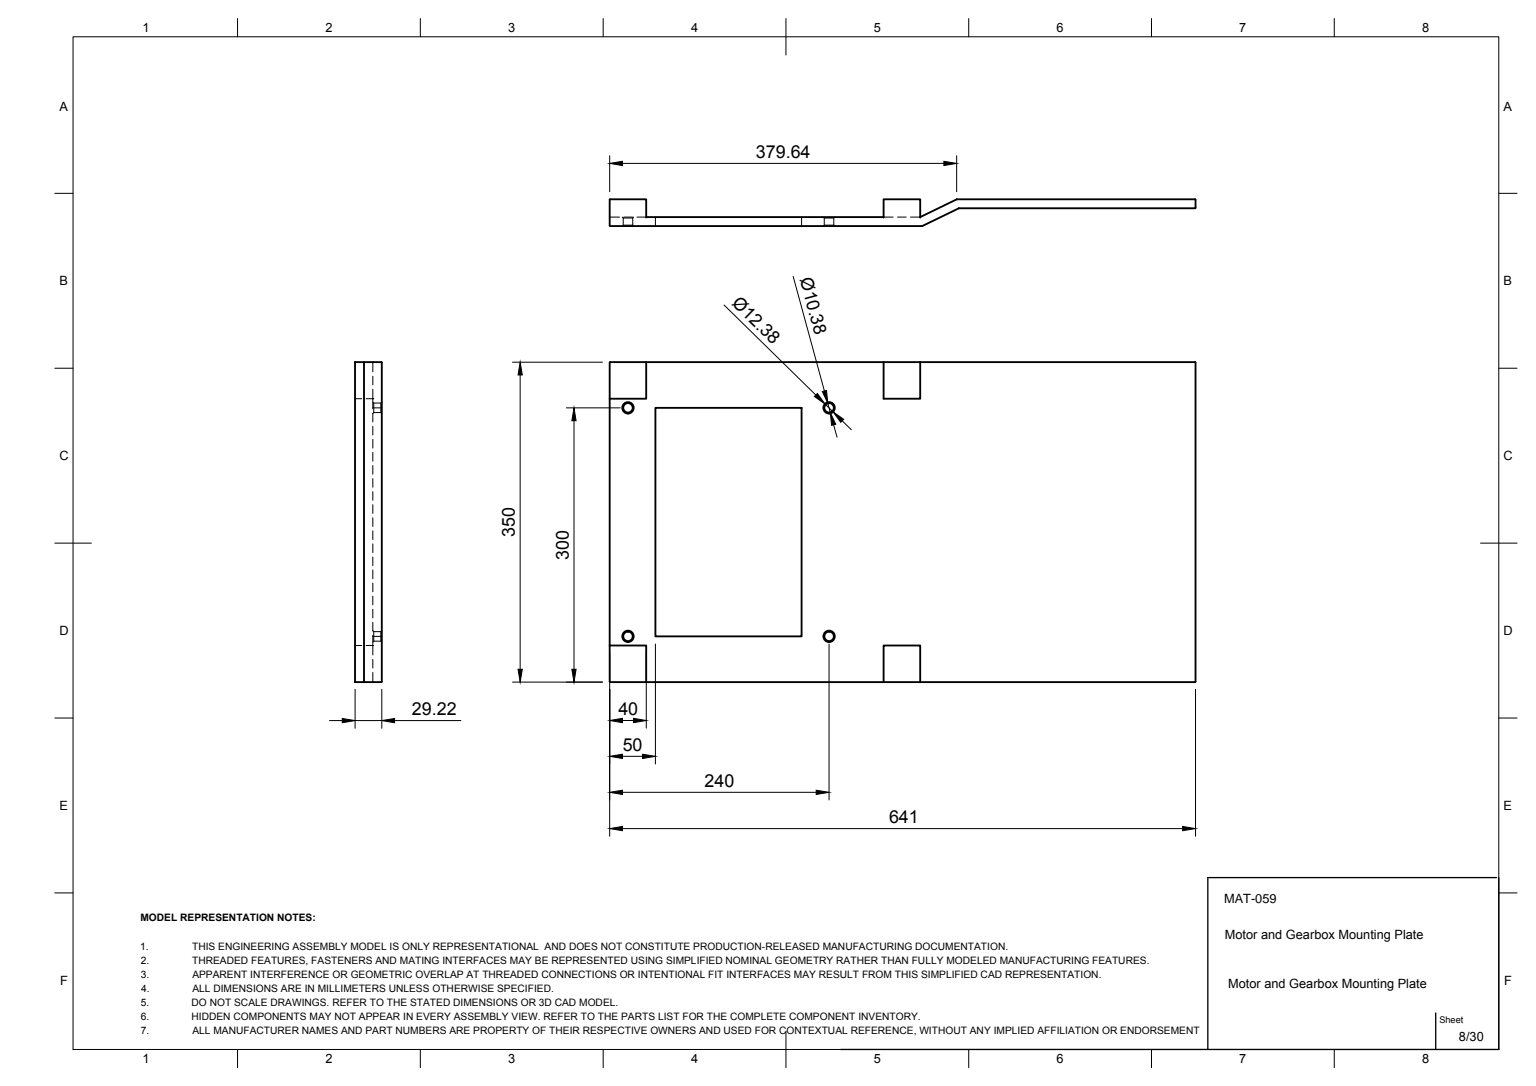
ISO-10303-21;
HEADER;
/* Generated by software containing ST-Developer
 * from STEP Tools, Inc. (www.steptools.com) 
 */

FILE_DESCRIPTION(
/* description */ ('', 'CAx-IF Rec.Pracs.---Representation and Presentation of Product Manufa
cturing Information (PMI)---4.0---2014-10-13'),
/* implementation_level */ '2;1');

FILE_NAME(
/* name */ 'Motor and Gearbox Mounting Plate.step',
/* time_stamp */ '2026-10-28T23:00:48+01:00',
/* author */ (''),
/* organization */ (''),
/* preprocessor_version */ 'ST-DEVELOPER v20.2',
/* originating_system */ 'Autodesk Translation Framework v15.17.0.0',
/* authorisation */ '');

FILE_SCHEMA (('AP242_MANAGED_MODEL_BASED_3D_ENGINEERING_MIM_LF { 1 0 10303 442 2 1 4 }'));
ENDSEC;

DATA;
#10=MECHANICAL_DESIGN_GEOMETRIC_PRESENTATION_REPRESENTATION('',(#970),#61811);
#390=ELLIPSE('',#35059,1.14442790218193,0.499999999899238);
#391=ELLIPSE('',#35060,1.14442790225741,0.499999999917943);
#392=ELLIPSE('',#35063,0.555857993550966,0.5);
#393=ELLIPSE('',#35139,0.555857993550966,0.5);
#474=B_SPLINE_SURFACE_WITH_KNOTS('',3,3,((#53444,#53445,#53446,#53447),
(#53448,#53449,#53450,#53451),(#53452,#53453,#53454,#53455),(#53456,#53457,
#53458,#53459)),.UNSPECIFIED.,.F.,.F.,.F.,(4,4),(4,4),(0.513291621409645,
1.),(-0.0253523930614869,0.),.UNSPECIFIED.);
#475=B_SPLINE_SURFACE_WITH_KNOTS('',3,3,((#53472,#53473,#53474,#53475),
(#53476,#53477,#53478,#53479),(#53480,#53481,#53482,#53483),(#53484,#53485,
#53486,#53487)),.UNSPECIFIED.,.F.,.F.,.F.,(4,4),(4,4),(0.513291621409645,
1.),(0.,0.0253730124676109),.UNSPECIFIED.);
#583=CONICAL_SURFACE('',#35152,5.68799999999971,0.785398163207466);
#584=CONICAL_SURFACE('',#35157,5.68799999999971,0.785398163337269);
#585=CONICAL_SURFACE('',#35162,5.68799999999971,0.785398163337269);
#586=CONICAL_SURFACE('',#35167,5.68799999999971,0.785398163207466);
#587=CONICAL_SURFACE('',#35172,5.688,0.785398163397448);
#588=CONICAL_SURFACE('',#35173,5.688,0.785398163397442);
#589=CONICAL_SURFACE('',#35174,5.688,0.785398163397442);
#590=CONICAL_SURFACE('',#35175,5.688,0.785398163397448);
#733=SPHERICAL_SURFACE('',#35068,0.499999999999998);
#734=SPHERICAL_SURFACE('',#35072,0.499999999999972);
#735=SPHERICAL_SURFACE('',#35076,0.499999999999972);
#736=SPHERICAL_SURFACE('',#35080,0.499999999999972);
#737=SPHERICAL_SURFACE('',#35084,0.499999999999998);
#738=SPHERICAL_SURFACE('',#35088,0.499999999999972);
#739=SPHERICAL_SURFACE('',#35101,0.5);
#740=SPHERICAL_SURFACE('',#35105,0.5);
#741=SPHERICAL_SURFACE('',#35112,0.499999999999998);
#742=SPHERICAL_SURFACE('',#35118,0.499999999999972);
#817=B_SPLINE_CURVE_WITH_KNOTS('',3,(#53461,#53462,#53463,#53464,#53465,
#53466,#53467,#53468,#53469,#53470),.UNSPECIFIED.,.F.,.F.,(4,2,2,2,4),(0.,
0.0127647979976817,0.0210777909778716,0.0238357493132096,0.025921076707915),
 .UNSPECIFIED.);
#818=B_SPLINE_CURVE_WITH_KNOTS('',3,(#53489,#53490,#53491,#53492,#53493,
#53494,#53495,#53496,#53497,#53498),.UNSPECIFIED.,.F.,.F.,(4,2,2,2,4),(0.,
0.00150625431059664,0.00349900031797075,0.00979302012528766,0.0186876936860384),
 .UNSPECIFIED.);
#896=TOROIDAL_SURFACE('',#35092,1.00000000000001,0.5);
#897=TOROIDAL_SURFACE('',#35097,1.,0.499999999999994);
#920=SHAPE_REPRESENTATION_RELATIONSHIP('SRR','None',#61978,#945);
#945=ADVANCED_BREP_SHAPE_REPRESENTATION('',(#1009),#61791);
#970=STYLED_ITEM('',(#62142),#1009);
#1009=MANIFOLD_SOLID_BREP('Body1',#33800);
#1163=CYLINDRICAL_SURFACE('',#35041,0.5);
#1164=CYLINDRICAL_SURFACE('',#35049,0.5);
#1165=CYLINDRICAL_SURFACE('',#35054,0.5);
#1166=CYLINDRICAL_SURFACE('',#35065,0.5);
#1167=CYLINDRICAL_SURFACE('',#35109,0.5);
#1168=CYLINDRICAL_SURFACE('',#35110,0.5);
#1169=CYLINDRICAL_SURFACE('',#35116,0.5);
#1170=CYLINDRICAL_SURFACE('',#35117,0.5);
#1171=CYLINDRICAL_SURFACE('',#35122,0.5);
#1172=CYLINDRICAL_SURFACE('',#35124,0.5);
#1173=CYLINDRICAL_SURFACE('',#35125,0.5);
#1174=CYLINDRICAL_SURFACE('',#35126,0.5);
#1175=CYLINDRICAL_SURFACE('',#35127,0.5);
#1176=CYLINDRICAL_SURFACE('',#35128,0.5);
#1177=CYLINDRICAL_SURFACE('',#35129,0.5);
#1178=CYLINDRICAL_SURFACE('',#35130,0.5);
#1179=CYLINDRICAL_SURFACE('',#35131,0.5);
#1180=CYLINDRICAL_SURFACE('',#35132,0.5);
#1181=CYLINDRICAL_SURFACE('',#35133,0.5);
#1182=CYLINDRICAL_SURFACE('',#35134,0.5);
#1183=CYLINDRICAL_SURFACE('',#35135,0.5);
#1184=CYLINDRICAL_SURFACE('',#35136,0.5);
#1185=CYLINDRICAL_SURFACE('',#35137,0.5);
#1186=CYLINDRICAL_SURFACE('',#35138,0.5);
#1187=CYLINDRICAL_SURFACE('',#35154,5.188);
#1188=CYLINDRICAL_SURFACE('',#35159,5.188);
#1189=CYLINDRICAL_SURFACE('',#35164,5.188);
#1190=CYLINDRICAL_SURFACE('',#35169,5.188);
#1968=FACE_BOUND('',#6698,.T.);
#1969=FACE_BOUND('',#6699,.T.);
#1970=FACE_BOUND('',#6700,.T.);
#1971=FACE_BOUND('',#6701,.T.);
#1972=FACE_BOUND('',#6702,.T.);
#1973=FACE_BOUND('',#6748,.T.);
#1974=FACE_BOUND('',#6749,.T.);
#1975=FACE_BOUND('',#6750,.T.);
#1976=FACE_BOUND('',#6751,.T.);
#1977=FACE_BOUND('',#6752,.T.);
#2674=CIRCLE('',#35042,0.5);
#2675=CIRCLE('',#35043,0.5);
#2676=CIRCLE('',#35045,6.188);
#2677=CIRCLE('',#35046,6.188);
#2678=CIRCLE('',#35047,6.188);
#2679=CIRCLE('',#35048,6.188);
#2680=CIRCLE('',#35050,0.5);
#2681=CIRCLE('',#35051,0.5);
#2682=CIRCLE('',#35053,1.00000000000015);
#2683=CIRCLE('',#35055,0.5);
#2684=CIRCLE('',#35056,0.5);
#2685=CIRCLE('',#35057,0.500000000000003);
#2686=CIRCLE('',#35058,0.499999999999992);
#2687=CIRCLE('',#35066,0.5);
#2688=CIRCLE('',#35067,0.5);
#2689=CIRCLE('',#35069,0.5);
#2690=CIRCLE('',#35070,0.499999999999998);
#2691=CIRCLE('',#35071,0.499999999999992);
#2692=CIRCLE('',#35073,0.499999999999998);
#2693=CIRCLE('',#35074,0.499999999999972);
#2694=CIRCLE('',#35075,0.499999999999996);
#2695=CIRCLE('',#35077,0.5);
#2696=CIRCLE('',#35078,0.499999999999972);
#2697=CIRCLE('',#35079,0.499999999999998);
#2698=CIRCLE('',#35081,0.499999999999972);
#2699=CIRCLE('',#35082,0.499999999999972);
#2700=CIRCLE('',#35083,0.499999999999998);
#2701=CIRCLE('',#35085,0.5);
#2702=CIRCLE('',#35086,0.499999999999998);
#2703=CIRCLE('',#35087,0.500000000000114);
#2704=CIRCLE('',#35089,0.499999999999998);
#2705=CIRCLE('',#35090,0.499999999999972);
#2706=CIRCLE('',#35091,0.499999999999972);
#2707=CIRCLE('',#35093,1.00000000000013);
#2708=CIRCLE('',#35094,0.500000000000006);
#2709=CIRCLE('',#35095,0.499999999999998);
#2710=CIRCLE('',#35096,0.5);
#2711=CIRCLE('',#35098,0.49999999999999);
#2712=CIRCLE('',#35099,0.499999999999972);
#2713=CIRCLE('',#35100,0.499999999999994);
#2714=CIRCLE('',#35102,0.5);
#2715=CIRCLE('',#35103,0.5);
#2716=CIRCLE('',#35104,0.500000000000002);
#2717=CIRCLE('',#35106,0.499999999999998);
#2718=CIRCLE('',#35107,0.5);
#2719=CIRCLE('',#35108,0.500000000000007);
#2720=CIRCLE('',#35111,0.5);
#2721=CIRCLE('',#35113,0.499999999999972);
#2722=CIRCLE('',#35114,0.499999999999998);
#2723=CIRCLE('',#35115,0.499999999999998);
#2724=CIRCLE('',#35119,0.500000000000007);
#2725=CIRCLE('',#35120,0.499999999999972);
#2726=CIRCLE('',#35121,0.500000000000003);
#2727=CIRCLE('',#35123,0.5);
#2728=CIRCLE('',#35144,6.18799999999941);
#2729=CIRCLE('',#35145,6.18799999999941);
#2730=CIRCLE('',#35146,6.18799999999941);
#2731=CIRCLE('',#35147,6.18799999999941);
#2732=CIRCLE('',#35153,5.188);
#2733=CIRCLE('',#35155,5.188);
#2734=CIRCLE('',#35156,5.188);
#2735=CIRCLE('',#35158,5.188);
#2736=CIRCLE('',#35160,5.188);
#2737=CIRCLE('',#35161,5.188);
#2738=CIRCLE('',#35163,5.188);
#2739=CIRCLE('',#35165,5.188);
#2740=CIRCLE('',#35166,5.188);
#2741=CIRCLE('',#35168,5.188);
#2742=CIRCLE('',#35170,5.188);
#2743=CIRCLE('',#35171,5.188);
#4728=FACE_OUTER_BOUND('',#6696,.T.);
#4729=FACE_OUTER_BOUND('',#6697,.T.);
#4730=FACE_OUTER_BOUND('',#6703,.T.);
#4731=FACE_OUTER_BOUND('',#6704,.T.);
#4732=FACE_OUTER_BOUND('',#6705,.T.);
#4733=FACE_OUTER_BOUND('',#6706,.T.);
#4734=FACE_OUTER_BOUND('',#6707,.T.);
#4735=FACE_OUTER_BOUND('',#6708,.T.);
#4736=FACE_OUTER_BOUND('',#6709,.T.);
#4737=FACE_OUTER_BOUND('',#6710,.T.);
#4738=FACE_OUTER_BOUND('',#6711,.T.);
#4739=FACE_OUTER_BOUND('',#6712,.T.);
#4740=FACE_OUTER_BOUND('',#6713,.T.);
#4741=FACE_OUTER_BOUND('',#6714,.T.);
#4742=FACE_OUTER_BOUND('',#6715,.T.);
#4743=FACE_OUTER_BOUND('',#6716,.T.);
#4744=FACE_OUTER_BOUND('',#6717,.T.);
#4745=FACE_OUTER_BOUND('',#6718,.T.);
#4746=FACE_OUTER_BOUND('',#6719,.T.);
#4747=FACE_OUTER_BOUND('',#6720,.T.);
#4748=FACE_OUTER_BOUND('',#6721,.T.);
#4749=FACE_OUTER_BOUND('',#6722,.T.);
#4750=FACE_OUTER_BOUND('',#6723,.T.);
#4751=FACE_OUTER_BOUND('',#6724,.T.);
#4752=FACE_OUTER_BOUND('',#6725,.T.);
#4753=FACE_OUTER_BOUND('',#6726,.T.);
#4754=FACE_OUTER_BOUND('',#6727,.T.);
#4755=FACE_OUTER_BOUND('',#6728,.T.);
#4756=FACE_OUTER_BOUND('',#6729,.T.);
#4757=FACE_OUTER_BOUND('',#6730,.T.);
#4758=FACE_OUTER_BOUND('',#6731,.T.);
#4759=FACE_OUTER_BOUND('',#6732,.T.);
#4760=FACE_OUTER_BOUND('',#6733,.T.);
#4761=FACE_OUTER_BOUND('',#6734,.T.);
#4762=FACE_OUTER_BOUND('',#6735,.T.);
#4763=FACE_OUTER_BOUND('',#6736,.T.);
#4764=FACE_OUTER_BOUND('',#6737,.T.);
#4765=FACE_OUTER_BOUND('',#6738,.T.);
#4766=FACE_OUTER_BOUND('',#6739,.T.);
#4767=FACE_OUTER_BOUND('',#6740,.T.);
#4768=FACE_OUTER_BOUND('',#6741,.T.);
#4769=FACE_OUTER_BOUND('',#6742,.T.);
#4770=FACE_OUTER_BOUND('',#6743,.T.);
#4771=FACE_OUTER_BOUND('',#6744,.T.);
#4772=FACE_OUTER_BOUND('',#6745,.T.);
#4773=FACE_OUTER_BOUND('',#6746,.T.);
#4774=FACE_OUTER_BOUND('',#6747,.T.);
#4775=FACE_OUTER_BOUND('',#6753,.T.);
#4776=FACE_OUTER_BOUND('',#6754,.T.);
#4777=FACE_OUTER_BOUND('',#6755,.T.);
#4778=FACE_OUTER_BOUND('',#6756,.T.);
#4779=FACE_OUTER_BOUND('',#6757,.T.);
#4780=FACE_OUTER_BOUND('',#6758,.T.);
#4781=FACE_OUTER_BOUND('',#6759,.T.);
#4782=FACE_OUTER_BOUND('',#6760,.T.);
#4783=FACE_OUTER_BOUND('',#6761,.T.);
#4784=FACE_OUTER_BOUND('',#6762,.T.);
#4785=FACE_OUTER_BOUND('',#6763,.T.);
#4786=FACE_OUTER_BOUND('',#6764,.T.);
#4787=FACE_OUTER_BOUND('',#6765,.T.);
#4788=FACE_OUTER_BOUND('',#6766,.T.);
#4789=FACE_OUTER_BOUND('',#6767,.T.);
#4790=FACE_OUTER_BOUND('',#6768,.T.);
#4791=FACE_OUTER_BOUND('',#6769,.T.);
#4792=FACE_OUTER_BOUND('',#6770,.T.);
#4793=FACE_OUTER_BOUND('',#6771,.T.);
#4794=FACE_OUTER_BOUND('',#6772,.T.);
#4795=FACE_OUTER_BOUND('',#6773,.T.);
#4796=FACE_OUTER_BOUND('',#6774,.T.);
#4797=FACE_OUTER_BOUND('',#6775,.T.);
#4798=FACE_OUTER_BOUND('',#6776,.T.);
#4799=FACE_OUTER_BOUND('',#6777,.T.);
#4800=FACE_OUTER_BOUND('',#6778,.T.);
#4801=FACE_OUTER_BOUND('',#6779,.T.);
#4802=FACE_OUTER_BOUND('',#6780,.T.);
#4803=FACE_OUTER_BOUND('',#6781,.T.);
#4804=FACE_OUTER_BOUND('',#6782,.T.);
#4805=FACE_OUTER_BOUND('',#6783,.T.);
#6696=EDGE_LOOP('',(#23838,#23839,#23840,#23841));
#6697=EDGE_LOOP('',(#23842,#23843,#23844,#23845,#23846,#23847,#23848,#23849,
#23850,#23851,#23852,#23853));
#6698=EDGE_LOOP('',(#23854));
#6699=EDGE_LOOP('',(#23855));
#6700=EDGE_LOOP('',(#23856,#23857,#23858,#23859));
#6701=EDGE_LOOP('',(#23860));
#6702=EDGE_LOOP('',(#23861));
#6703=EDGE_LOOP('',(#23862,#23863,#23864,#23865));
#6704=EDGE_LOOP('',(#23866,#23867,#23868,#23869,#23870,#23871,#23872,#23873,
#23874,#23875,#23876,#23877,#23878,#23879));
#6705=EDGE_LOOP('',(#23880,#23881,#23882,#23883,#23884,#23885));
#6706=EDGE_LOOP('',(#23886,#23887,#23888));
#6707=EDGE_LOOP('',(#23889,#23890,#23891));
#6708=EDGE_LOOP('',(#23892,#23893,#23894,#23895,#23896));
#6709=EDGE_LOOP('',(#23897,#23898,#23899,#23900,#23901,#23902));
#6710=EDGE_LOOP('',(#23903,#23904,#23905,#23906,#23907,#23908,#23909,#23910));
#6711=EDGE_LOOP('',(#23911,#23912,#23913,#23914));
#6712=EDGE_LOOP('',(#23915,#23916,#23917));
#6713=EDGE_LOOP('',(#23918,#23919,#23920));
#6714=EDGE_LOOP('',(#23921,#23922,#23923));
#6715=EDGE_LOOP('',(#23924,#23925,#23926));
#6716=EDGE_LOOP('',(#23927,#23928,#23929));
#6717=EDGE_LOOP('',(#23930,#23931,#23932));
#6718=EDGE_LOOP('',(#23933,#23934,#23935,#23936));
#6719=EDGE_LOOP('',(#23937,#23938,#23939,#23940));
#6720=EDGE_LOOP('',(#23941,#23942,#23943));
#6721=EDGE_LOOP('',(#23944,#23945,#23946));
#6722=EDGE_LOOP('',(#23947,#23948,#23949,#23950));
#6723=EDGE_LOOP('',(#23951,#23952,#23953,#23954));
#6724=EDGE_LOOP('',(#23955,#23956,#23957));
#6725=EDGE_LOOP('',(#23958,#23959,#23960,#23961));
#6726=EDGE_LOOP('',(#23962,#23963,#23964,#23965));
#6727=EDGE_LOOP('',(#23966,#23967,#23968));
#6728=EDGE_LOOP('',(#23969,#23970,#23971,#23972));
#6729=EDGE_LOOP('',(#23973,#23974,#23975,#23976));
#6730=EDGE_LOOP('',(#23977,#23978,#23979,#23980));
#6731=EDGE_LOOP('',(#23981,#23982,#23983,#23984));
#6732=EDGE_LOOP('',(#23985,#23986,#23987,#23988));
#6733=EDGE_LOOP('',(#23989,#23990,#23991,#23992));
#6734=EDGE_LOOP('',(#23993,#23994,#23995,#23996));
#6735=EDGE_LOOP('',(#23997,#23998,#23999,#24000));
#6736=EDGE_LOOP('',(#24001,#24002,#24003,#24004));
#6737=EDGE_LOOP('',(#24005,#24006,#24007,#24008));
#6738=EDGE_LOOP('',(#24009,#24010,#24011,#24012));
#6739=EDGE_LOOP('',(#24013,#24014,#24015,#24016));
#6740=EDGE_LOOP('',(#24017,#24018,#24019,#24020));
#6741=EDGE_LOOP('',(#24021,#24022,#24023,#24024));
#6742=EDGE_LOOP('',(#24025,#24026,#24027,#24028));
#6743=EDGE_LOOP('',(#24029,#24030,#24031,#24032));
#6744=EDGE_LOOP('',(#24033,#24034,#24035,#24036,#24037,#24038,#24039,#24040));
#6745=EDGE_LOOP('',(#24041,#24042,#24043,#24044,#24045));
#6746=EDGE_LOOP('',(#24046,#24047,#24048,#24049,#24050,#24051,#24052,#24053,
#24054,#24055,#24056,#24057,#24058,#24059));
#6747=EDGE_LOOP('',(#24060,#24061,#24062,#24063));
#6748=EDGE_LOOP('',(#24064));
#6749=EDGE_LOOP('',(#24065));
#6750=EDGE_LOOP('',(#24066,#24067,#24068,#24069));
#6751=EDGE_LOOP('',(#24070));
#6752=EDGE_LOOP('',(#24071));
#6753=EDGE_LOOP('',(#24072,#24073,#24074,#24075));
#6754=EDGE_LOOP('',(#24076,#24077,#24078,#24079));
#6755=EDGE_LOOP('',(#24080,#24081,#24082,#24083));
#6756=EDGE_LOOP('',(#24084,#24085,#24086,#24087));
#6757=EDGE_LOOP('',(#24088,#24089,#24090,#24091));
#6758=EDGE_LOOP('',(#24092,#24093,#24094,#24095,#24096));
#6759=EDGE_LOOP('',(#24097,#24098,#24099,#24100));
#6760=EDGE_LOOP('',(#24101,#24102,#24103,#24104,#24105));
#6761=EDGE_LOOP('',(#24106,#24107,#24108,#24109));
#6762=EDGE_LOOP('',(#24110,#24111,#24112,#24113,#24114));
#6763=EDGE_LOOP('',(#24115,#24116,#24117,#24118));
#6764=EDGE_LOOP('',(#24119,#24120,#24121,#24122,#24123));
#6765=EDGE_LOOP('',(#24124,#24125,#24126,#24127,#24128));
#6766=EDGE_LOOP('',(#24129,#24130,#24131,#24132,#24133));
#6767=EDGE_LOOP('',(#24134,#24135,#24136,#24137,#24138));
#6768=EDGE_LOOP('',(#24139,#24140,#24141,#24142,#24143));
#6769=EDGE_LOOP('',(#24144,#24145,#24146,#24147,#24148));
#6770=EDGE_LOOP('',(#24149,#24150,#24151,#24152,#24153));
#6771=EDGE_LOOP('',(#24154,#24155,#24156,#24157));
#6772=EDGE_LOOP('',(#24158,#24159,#24160,#24161,#24162));
#6773=EDGE_LOOP('',(#24163,#24164,#24165,#24166,#24167,#24168));
#6774=EDGE_LOOP('',(#24169,#24170,#24171,#24172,#24173));
#6775=EDGE_LOOP('',(#24174,#24175,#24176,#24177,#24178));
#6776=EDGE_LOOP('',(#24179,#24180,#24181,#24182,#24183));
#6777=EDGE_LOOP('',(#24184,#24185,#24186,#24187,#24188));
#6778=EDGE_LOOP('',(#24189,#24190,#24191,#24192));
#6779=EDGE_LOOP('',(#24193,#24194,#24195,#24196,#24197));
#6780=EDGE_LOOP('',(#24198,#24199,#24200,#24201));
#6781=EDGE_LOOP('',(#24202,#24203,#24204,#24205));
#6782=EDGE_LOOP('',(#24206,#24207,#24208,#24209));
#6783=EDGE_LOOP('',(#24210,#24211,#24212,#24213));
#8989=LINE('',#53360,#11536);
#8990=LINE('',#53363,#11537);
#8991=LINE('',#53366,#11538);
#8992=LINE('',#53368,#11539);
#8993=LINE('',#53370,#11540);
#8994=LINE('',#53372,#11541);
#8995=LINE('',#53374,#11542);
#8996=LINE('',#53376,#11543);
#8997=LINE('',#53378,#11544);
#8998=LINE('',#53380,#11545);
#8999=LINE('',#53382,#11546);
#9000=LINE('',#53384,#11547);
#9001=LINE('',#53385,#11548);
#9002=LINE('',#53392,#11549);
#9003=LINE('',#53394,#11550);
#9004=LINE('',#53396,#11551);
#9005=LINE('',#53397,#11552);
#9006=LINE('',#53406,#11553);
#9007=LINE('',#53410,#11554);
#9008=LINE('',#53412,#11555);
#9009=LINE('',#53414,#11556);
#9010=LINE('',#53416,#11557);
#9011=LINE('',#53418,#11558);
#9012=LINE('',#53420,#11559);
#9013=LINE('',#53422,#11560);
#9014=LINE('',#53424,#11561);
#9015=LINE('',#53428,#11562);
#9016=LINE('',#53430,#11563);
#9017=LINE('',#53432,#11564);
#9018=LINE('',#53433,#11565);
#9019=LINE('',#53442,#11566);
#9020=LINE('',#53502,#11567);
#9021=LINE('',#53504,#11568);
#9022=LINE('',#53505,#11569);
#9023=LINE('',#53508,#11570);
#9024=LINE('',#53510,#11571);
#9025=LINE('',#53513,#11572);
#9026=LINE('',#53515,#11573);
#9027=LINE('',#53517,#11574);
#9028=LINE('',#53518,#11575);
#9029=LINE('',#53524,#11576);
#9030=LINE('',#53592,#11577);
#9031=LINE('',#53593,#11578);
#9032=LINE('',#53598,#11579);
#9033=LINE('',#53599,#11580);
#9034=LINE('',#53607,#11581);
#9035=LINE('',#53609,#11582);
#9036=LINE('',#53610,#11583);
#9037=LINE('',#53620,#11584);
#9038=LINE('',#53622,#11585);
#9039=LINE('',#53624,#11586);
#9040=LINE('',#53625,#11587);
#9041=LINE('',#53627,#11588);
#9042=LINE('',#53628,#11589);
#9043=LINE('',#53630,#11590);
#9044=LINE('',#53632,#11591);
#9045=LINE('',#53633,#11592);
#9046=LINE('',#53635,#11593);
#9047=LINE('',#53636,#11594);
#9048=LINE('',#53638,#11595);
#9049=LINE('',#53640,#11596);
#9050=LINE('',#53641,#11597);
#9051=LINE('',#53643,#11598);
#9052=LINE('',#53644,#11599);
#9053=LINE('',#53646,#11600);
#9054=LINE('',#53648,#11601);
#9055=LINE('',#53649,#11602);
#9056=LINE('',#53651,#11603);
#9057=LINE('',#53652,#11604);
#9058=LINE('',#53655,#11605);
#9059=LINE('',#53659,#11606);
#9060=LINE('',#53662,#11607);
#9061=LINE('',#53663,#11608);
#9062=LINE('',#53665,#11609);
#9063=LINE('',#53666,#11610);
#9064=LINE('',#53669,#11611);
#9065=LINE('',#53671,#11612);
#9066=LINE('',#53672,#11613);
#9067=LINE('',#53674,#11614);
#9068=LINE('',#53676,#11615);
#9069=LINE('',#53678,#11616);
#9070=LINE('',#53679,#11617);
#9071=LINE('',#53687,#11618);
#9072=LINE('',#53689,#11619);
#9073=LINE('',#53691,#11620);
#9074=LINE('',#53692,#11621);
#9075=LINE('',#53704,#11622);
#9076=LINE('',#53707,#11623);
#9077=LINE('',#53714,#11624);
#9078=LINE('',#53717,#11625);
#9079=LINE('',#53724,#11626);
#9080=LINE('',#53727,#11627);
#9081=LINE('',#53734,#11628);
#9082=LINE('',#53737,#11629);
#9083=LINE('',#53742,#11630);
#9084=LINE('',#53744,#11631);
#9085=LINE('',#53746,#11632);
#9086=LINE('',#53748,#11633);
#9087=LINE('',#53750,#11634);
#9088=LINE('',#53754,#11635);
#9089=LINE('',#53756,#11636);
#9090=LINE('',#53757,#11637);
#9091=LINE('',#53759,#11638);
#9092=LINE('',#53761,#11639);
#9093=LINE('',#53765,#11640);
#9094=LINE('',#53766,#11641);
#9095=LINE('',#53768,#11642);
#9096=LINE('',#53771,#11643);
#9097=LINE('',#53774,#11644);
#9098=LINE('',#53775,#11645);
#9099=LINE('',#53777,#11646);
#9100=LINE('',#53779,#11647);
#11536=VECTOR('',#40671,10.);
#11537=VECTOR('',#40674,10.);
#11538=VECTOR('',#40677,10.);
#11539=VECTOR('',#40678,10.);
#11540=VECTOR('',#40679,10.);
#11541=VECTOR('',#40680,10.);
#11542=VECTOR('',#40681,10.);
#11543=VECTOR('',#40682,10.);
#11544=VECTOR('',#40683,10.);
#11545=VECTOR('',#40684,10.);
#11546=VECTOR('',#40685,10.);
#11547=VECTOR('',#40686,10.);
#11548=VECTOR('',#40687,10.);
#11549=VECTOR('',#40692,10.);
#11550=VECTOR('',#40693,10.);
#11551=VECTOR('',#40694,10.);
#11552=VECTOR('',#40695,10.);
#11553=VECTOR('',#40704,10.);
#11554=VECTOR('',#40709,10.);
#11555=VECTOR('',#40710,10.);
#11556=VECTOR('',#40711,10.);
#11557=VECTOR('',#40712,10.);
#11558=VECTOR('',#40713,10.);
#11559=VECTOR('',#40714,10.);
#11560=VECTOR('',#40715,10.);
#11561=VECTOR('',#40716,10.);
#11562=VECTOR('',#40719,10.);
#11563=VECTOR('',#40720,10.);
#11564=VECTOR('',#40721,10.);
#11565=VECTOR('',#40722,10.);
#11566=VECTOR('',#40731,10.);
#11567=VECTOR('',#40740,10.);
#11568=VECTOR('',#40741,10.);
#11569=VECTOR('',#40742,10.);
#11570=VECTOR('',#40745,10.);
#11571=VECTOR('',#40748,10.);
#11572=VECTOR('',#40751,10.);
#11573=VECTOR('',#40752,10.);
#11574=VECTOR('',#40753,10.);
#11575=VECTOR('',#40754,10.);
#11576=VECTOR('',#40761,10.);
#11577=VECTOR('',#40846,10.);
#11578=VECTOR('',#40847,10.);
#11579=VECTOR('',#40852,10.);
#11580=VECTOR('',#40853,10.);
#11581=VECTOR('',#40864,10.);
#11582=VECTOR('',#40867,10.);
#11583=VECTOR('',#40868,10.);
#11584=VECTOR('',#40881,10.);
#11585=VECTOR('',#40884,10.);
#11586=VECTOR('',#40887,10.);
#11587=VECTOR('',#40888,10.);
#11588=VECTOR('',#40891,10.);
#11589=VECTOR('',#40892,10.);
#11590=VECTOR('',#40895,10.);
#11591=VECTOR('',#40898,10.);
#11592=VECTOR('',#40899,10.);
#11593=VECTOR('',#40902,10.);
#11594=VECTOR('',#40903,10.);
#11595=VECTOR('',#40906,10.);
#11596=VECTOR('',#40909,10.);
#11597=VECTOR('',#40910,10.);
#11598=VECTOR('',#40913,10.);
#11599=VECTOR('',#40914,10.);
#11600=VECTOR('',#40917,10.);
#11601=VECTOR('',#40920,10.);
#11602=VECTOR('',#40921,10.);
#11603=VECTOR('',#40924,10.);
#11604=VECTOR('',#40925,10.);
#11605=VECTOR('',#40930,10.);
#11606=VECTOR('',#40935,10.);
#11607=VECTOR('',#40938,10.);
#11608=VECTOR('',#40939,10.);
#11609=VECTOR('',#40940,10.);
#11610=VECTOR('',#40941,10.);
#11611=VECTOR('',#40944,10.);
#11612=VECTOR('',#40945,10.);
#11613=VECTOR('',#40946,10.);
#11614=VECTOR('',#40949,10.);
#11615=VECTOR('',#40950,10.);
#11616=VECTOR('',#40951,10.);
#11617=VECTOR('',#40952,10.);
#11618=VECTOR('',#40959,10.);
#11619=VECTOR('',#40960,10.);
#11620=VECTOR('',#40961,10.);
#11621=VECTOR('',#40962,10.);
#11622=VECTOR('',#40979,5.68799999999971);
#11623=VECTOR('',#40982,5.188);
#11624=VECTOR('',#40991,5.68799999999971);
#11625=VECTOR('',#40994,5.188);
#11626=VECTOR('',#41003,5.68799999999971);
#11627=VECTOR('',#41006,5.188);
#11628=VECTOR('',#41015,5.68799999999971);
#11629=VECTOR('',#41018,5.188);
#11630=VECTOR('',#41025,5.688);
#11631=VECTOR('',#41028,5.688);
#11632=VECTOR('',#41031,5.688);
#11633=VECTOR('',#41034,5.688);
#11634=VECTOR('',#41037,10.);
#11635=VECTOR('',#41042,10.);
#11636=VECTOR('',#41043,10.);
#11637=VECTOR('',#41044,10.);
#11638=VECTOR('',#41047,10.);
#11639=VECTOR('',#41050,10.);
#11640=VECTOR('',#41055,10.);
#11641=VECTOR('',#41056,10.);
#11642=VECTOR('',#41059,10.);
#11643=VECTOR('',#41064,10.);
#11644=VECTOR('',#41069,10.);
#11645=VECTOR('',#41070,10.);
#11646=VECTOR('',#41073,10.);
#11647=VECTOR('',#41076,10.);
#14210=VERTEX_POINT('',#53356);
#14211=VERTEX_POINT('',#53357);
#14212=VERTEX_POINT('',#53359);
#14213=VERTEX_POINT('',#53361);
#14214=VERTEX_POINT('',#53365);
#14215=VERTEX_POINT('',#53367);
#14216=VERTEX_POINT('',#53369);
#14217=VERTEX_POINT('',#53371);
#14218=VERTEX_POINT('',#53373);
#14219=VERTEX_POINT('',#53375);
#14220=VERTEX_POINT('',#53377);
#14221=VERTEX_POINT('',#53379);
#14222=VERTEX_POINT('',#53381);
#14223=VERTEX_POINT('',#53383);
#14224=VERTEX_POINT('',#53386);
#14225=VERTEX_POINT('',#53388);
#14226=VERTEX_POINT('',#53390);
#14227=VERTEX_POINT('',#53391);
#14228=VERTEX_POINT('',#53393);
#14229=VERTEX_POINT('',#53395);
#14230=VERTEX_POINT('',#53398);
#14231=VERTEX_POINT('',#53400);
#14232=VERTEX_POINT('',#53403);
#14233=VERTEX_POINT('',#53405);
#14234=VERTEX_POINT('',#53409);
#14235=VERTEX_POINT('',#53411);
#14236=VERTEX_POINT('',#53413);
#14237=VERTEX_POINT('',#53415);
#14238=VERTEX_POINT('',#53417);
#14239=VERTEX_POINT('',#53419);
#14240=VERTEX_POINT('',#53421);
#14241=VERTEX_POINT('',#53423);
#14242=VERTEX_POINT('',#53425);
#14243=VERTEX_POINT('',#53427);
#14244=VERTEX_POINT('',#53429);
#14245=VERTEX_POINT('',#53431);
#14246=VERTEX_POINT('',#53435);
#14247=VERTEX_POINT('',#53437);
#14248=VERTEX_POINT('',#53439);
#14249=VERTEX_POINT('',#53441);
#14250=VERTEX_POINT('',#53460);
#14251=VERTEX_POINT('',#53488);
#14252=VERTEX_POINT('',#53501);
#14253=VERTEX_POINT('',#53503);
#14254=VERTEX_POINT('',#53507);
#14255=VERTEX_POINT('',#53512);
#14256=VERTEX_POINT('',#53514);
#14257=VERTEX_POINT('',#53516);
#14258=VERTEX_POINT('',#53520);
#14259=VERTEX_POINT('',#53522);
#14260=VERTEX_POINT('',#53526);
#14261=VERTEX_POINT('',#53528);
#14262=VERTEX_POINT('',#53532);
#14263=VERTEX_POINT('',#53537);
#14264=VERTEX_POINT('',#53538);
#14265=VERTEX_POINT('',#53540);
#14266=VERTEX_POINT('',#53544);
#14267=VERTEX_POINT('',#53545);
#14268=VERTEX_POINT('',#53550);
#14269=VERTEX_POINT('',#53551);
#14270=VERTEX_POINT('',#53553);
#14271=VERTEX_POINT('',#53557);
#14272=VERTEX_POINT('',#53558);
#14273=VERTEX_POINT('',#53563);
#14274=VERTEX_POINT('',#53564);
#14275=VERTEX_POINT('',#53566);
#14276=VERTEX_POINT('',#53568);
#14277=VERTEX_POINT('',#53572);
#14278=VERTEX_POINT('',#53573);
#14279=VERTEX_POINT('',#53578);
#14280=VERTEX_POINT('',#53579);
#14281=VERTEX_POINT('',#53581);
#14282=VERTEX_POINT('',#53585);
#14283=VERTEX_POINT('',#53586);
#14284=VERTEX_POINT('',#53588);
#14285=VERTEX_POINT('',#53595);
#14286=VERTEX_POINT('',#53596);
#14287=VERTEX_POINT('',#53601);
#14288=VERTEX_POINT('',#53603);
#14289=VERTEX_POINT('',#53612);
#14290=VERTEX_POINT('',#53613);
#14291=VERTEX_POINT('',#53618);
#14292=VERTEX_POINT('',#53657);
#14293=VERTEX_POINT('',#53661);
#14294=VERTEX_POINT('',#53664);
#14295=VERTEX_POINT('',#53668);
#14296=VERTEX_POINT('',#53670);
#14297=VERTEX_POINT('',#53675);
#14298=VERTEX_POINT('',#53677);
#14299=VERTEX_POINT('',#53681);
#14300=VERTEX_POINT('',#53683);
#14301=VERTEX_POINT('',#53685);
#14302=VERTEX_POINT('',#53686);
#14303=VERTEX_POINT('',#53688);
#14304=VERTEX_POINT('',#53690);
#14305=VERTEX_POINT('',#53693);
#14306=VERTEX_POINT('',#53695);
#14307=VERTEX_POINT('',#53702);
#14308=VERTEX_POINT('',#53706);
#14309=VERTEX_POINT('',#53708);
#14310=VERTEX_POINT('',#53712);
#14311=VERTEX_POINT('',#53716);
#14312=VERTEX_POINT('',#53718);
#14313=VERTEX_POINT('',#53722);
#14314=VERTEX_POINT('',#53726);
#14315=VERTEX_POINT('',#53728);
#14316=VERTEX_POINT('',#53732);
#14317=VERTEX_POINT('',#53736);
#14318=VERTEX_POINT('',#53738);
#14319=VERTEX_POINT('',#53753);
#14320=VERTEX_POINT('',#53755);
#14321=VERTEX_POINT('',#53764);
#17821=EDGE_CURVE('',#14210,#14211,#2674,.F.);
#17822=EDGE_CURVE('',#14211,#14212,#8989,.T.);
#17823=EDGE_CURVE('',#14212,#14213,#2675,.F.);
#17824=EDGE_CURVE('',#14213,#14210,#8990,.T.);
#17825=EDGE_CURVE('',#14211,#14214,#8991,.T.);
#17826=EDGE_CURVE('',#14214,#14215,#8992,.T.);
#17827=EDGE_CURVE('',#14216,#14215,#8993,.T.);
#17828=EDGE_CURVE('',#14216,#14217,#8994,.T.);
#17829=EDGE_CURVE('',#14217,#14218,#8995,.T.);
#17830=EDGE_CURVE('',#14219,#14218,#8996,.T.);
#17831=EDGE_CURVE('',#14219,#14220,#8997,.T.);
#17832=EDGE_CURVE('',#14220,#14221,#8998,.T.);
#17833=EDGE_CURVE('',#14222,#14221,#8999,.T.);
#17834=EDGE_CURVE('',#14222,#14223,#9000,.T.);
#17835=EDGE_CURVE('',#14223,#14212,#9001,.T.);
#17836=EDGE_CURVE('',#14224,#14224,#2676,.T.);
#17837=EDGE_CURVE('',#14225,#14225,#2677,.T.);
#17838=EDGE_CURVE('',#14226,#14227,#9002,.T.);
#17839=EDGE_CURVE('',#14227,#14228,#9003,.T.);
#17840=EDGE_CURVE('',#14228,#14229,#9004,.T.);
#17841=EDGE_CURVE('',#14229,#14226,#9005,.T.);
#17842=EDGE_CURVE('',#14230,#14230,#2678,.T.);
#17843=EDGE_CURVE('',#14231,#14231,#2679,.T.);
#17844=EDGE_CURVE('',#14221,#14232,#2680,.F.);
#17845=EDGE_CURVE('',#14232,#14233,#9006,.T.);
#17846=EDGE_CURVE('',#14233,#14222,#2681,.F.);
#17847=EDGE_CURVE('',#14233,#14234,#9007,.T.);
#17848=EDGE_CURVE('',#14232,#14235,#9008,.T.);
#17849=EDGE_CURVE('',#14235,#14236,#9009,.T.);
#17850=EDGE_CURVE('',#14237,#14236,#9010,.T.);
#17851=EDGE_CURVE('',#14238,#14237,#9011,.T.);
#17852=EDGE_CURVE('',#14239,#14238,#9012,.T.);
#17853=EDGE_CURVE('',#14240,#14239,#9013,.T.);
#17854=EDGE_CURVE('',#14241,#14240,#9014,.T.);
#17855=EDGE_CURVE('',#14242,#14241,#2682,.T.);
#17856=EDGE_CURVE('',#14243,#14242,#9015,.T.);
#17857=EDGE_CURVE('',#14244,#14243,#9016,.T.);
#17858=EDGE_CURVE('',#14245,#14244,#9017,.T.);
#17859=EDGE_CURVE('',#14245,#14234,#9018,.T.);
#17860=EDGE_CURVE('',#14219,#14246,#2683,.T.);
#17861=EDGE_CURVE('',#14247,#14218,#2684,.T.);
#17862=EDGE_CURVE('',#14247,#14248,#2685,.T.);
#17863=EDGE_CURVE('',#14248,#14249,#9019,.T.);
#17864=EDGE_CURVE('',#14249,#14246,#2686,.T.);
#17865=EDGE_CURVE('',#14250,#14247,#817,.T.);
#17866=EDGE_CURVE('',#14250,#14248,#390,.T.);
#17867=EDGE_CURVE('',#14246,#14251,#818,.T.);
#17868=EDGE_CURVE('',#14249,#14251,#391,.T.);
#17869=EDGE_CURVE('',#14246,#14252,#9020,.T.);
#17870=EDGE_CURVE('',#14252,#14253,#9021,.T.);
#17871=EDGE_CURVE('',#14220,#14253,#9022,.T.);
#17872=EDGE_CURVE('',#14251,#14254,#9023,.T.);
#17873=EDGE_CURVE('',#14237,#14254,#392,.F.);
#17874=EDGE_CURVE('',#14236,#14252,#9024,.T.);
#17875=EDGE_CURVE('',#14255,#14250,#9025,.T.);
#17876=EDGE_CURVE('',#14256,#14255,#9026,.T.);
#17877=EDGE_CURVE('',#14257,#14256,#9027,.T.);
#17878=EDGE_CURVE('',#14254,#14257,#9028,.T.);
#17879=EDGE_CURVE('',#14258,#14216,#2687,.F.);
#17880=EDGE_CURVE('',#14215,#14259,#2688,.F.);
#17881=EDGE_CURVE('',#14259,#14258,#9029,.T.);
#17882=EDGE_CURVE('',#14260,#14256,#2689,.F.);
#17883=EDGE_CURVE('',#14261,#14260,#2690,.F.);
#17884=EDGE_CURVE('',#14256,#14261,#2691,.F.);
#17885=EDGE_CURVE('',#14262,#14257,#2692,.F.);
#17886=EDGE_CURVE('',#14238,#14262,#2693,.F.);
#17887=EDGE_CURVE('',#14257,#14238,#2694,.F.);
#17888=EDGE_CURVE('',#14263,#14264,#2695,.F.);
#17889=EDGE_CURVE('',#14265,#14263,#2696,.F.);
#17890=EDGE_CURVE('',#14264,#14265,#2697,.F.);
#17891=EDGE_CURVE('',#14266,#14267,#2698,.F.);
#17892=EDGE_CURVE('',#14239,#14266,#2699,.F.);
#17893=EDGE_CURVE('',#14267,#14239,#2700,.F.);
#17894=EDGE_CURVE('',#14268,#14269,#2701,.F.);
#17895=EDGE_CURVE('',#14270,#14268,#2702,.F.);
#17896=EDGE_CURVE('',#14269,#14270,#2703,.F.);
#17897=EDGE_CURVE('',#14271,#14272,#2704,.F.);
#17898=EDGE_CURVE('',#14240,#14271,#2705,.F.);
#17899=EDGE_CURVE('',#14272,#14240,#2706,.F.);
#17900=EDGE_CURVE('',#14273,#14274,#2707,.T.);
#17901=EDGE_CURVE('',#14275,#14274,#2708,.T.);
#17902=EDGE_CURVE('',#14276,#14275,#2709,.F.);
#17903=EDGE_CURVE('',#14273,#14276,#2710,.T.);
#17904=EDGE_CURVE('',#14277,#14278,#2711,.F.);
#17905=EDGE_CURVE('',#14242,#14277,#2712,.T.);
#17906=EDGE_CURVE('',#14278,#14241,#2713,.T.);
#17907=EDGE_CURVE('',#14279,#14280,#2714,.F.);
#17908=EDGE_CURVE('',#14281,#14279,#2715,.F.);
#17909=EDGE_CURVE('',#14280,#14281,#2716,.F.);
#17910=EDGE_CURVE('',#14282,#14283,#2717,.F.);
#17911=EDGE_CURVE('',#14284,#14282,#2718,.F.);
#17912=EDGE_CURVE('',#14283,#14284,#2719,.F.);
#17913=EDGE_CURVE('',#14279,#14284,#9030,.T.);
#17914=EDGE_CURVE('',#14282,#14281,#9031,.T.);
#17915=EDGE_CURVE('',#14285,#14286,#2720,.T.);
#17916=EDGE_CURVE('',#14286,#14283,#9032,.T.);
#17917=EDGE_CURVE('',#14284,#14285,#9033,.T.);
#17918=EDGE_CURVE('',#14243,#14287,#2721,.F.);
#17919=EDGE_CURVE('',#14288,#14243,#2722,.F.);
#17920=EDGE_CURVE('',#14287,#14288,#2723,.F.);
#17921=EDGE_CURVE('',#14277,#14288,#9034,.T.);
#17922=EDGE_CURVE('',#14288,#14280,#9035,.T.);
#17923=EDGE_CURVE('',#14281,#14287,#9036,.T.);
#17924=EDGE_CURVE('',#14289,#14290,#2724,.F.);
#17925=EDGE_CURVE('',#14244,#14289,#2725,.F.);
#17926=EDGE_CURVE('',#14290,#14244,#2726,.F.);
#17927=EDGE_CURVE('',#14291,#14245,#2727,.T.);
#17928=EDGE_CURVE('',#14289,#14291,#9037,.T.);
#17929=EDGE_CURVE('',#14287,#14290,#9038,.T.);
#17930=EDGE_CURVE('',#14290,#14282,#9039,.T.);
#17931=EDGE_CURVE('',#14283,#14289,#9040,.T.);
#17932=EDGE_CURVE('',#14274,#14279,#9041,.T.);
#17933=EDGE_CURVE('',#14280,#14275,#9042,.T.);
#17934=EDGE_CURVE('',#14271,#14278,#9043,.T.);
#17935=EDGE_CURVE('',#14278,#14276,#9044,.T.);
#17936=EDGE_CURVE('',#14275,#14277,#9045,.T.);
#17937=EDGE_CURVE('',#14268,#14273,#9046,.T.);
#17938=EDGE_CURVE('',#14276,#14270,#9047,.T.);
#17939=EDGE_CURVE('',#14266,#14272,#9048,.T.);
#17940=EDGE_CURVE('',#14272,#14269,#9049,.T.);
#17941=EDGE_CURVE('',#14270,#14271,#9050,.T.);
#17942=EDGE_CURVE('',#14263,#14268,#9051,.T.);
#17943=EDGE_CURVE('',#14269,#14265,#9052,.T.);
#17944=EDGE_CURVE('',#14262,#14267,#9053,.T.);
#17945=EDGE_CURVE('',#14267,#14264,#9054,.T.);
#17946=EDGE_CURVE('',#14265,#14266,#9055,.T.);
#17947=EDGE_CURVE('',#14260,#14263,#9056,.T.);
#17948=EDGE_CURVE('',#14264,#14261,#9057,.T.);
#17949=EDGE_CURVE('',#14261,#14262,#9058,.T.);
#17950=EDGE_CURVE('',#14255,#14292,#393,.F.);
#17951=EDGE_CURVE('',#14292,#14260,#9059,.T.);
#17952=EDGE_CURVE('',#14213,#14293,#9060,.T.);
#17953=EDGE_CURVE('',#14293,#14291,#9061,.T.);
#17954=EDGE_CURVE('',#14286,#14294,#9062,.T.);
#17955=EDGE_CURVE('',#14210,#14294,#9063,.T.);
#17956=EDGE_CURVE('',#14295,#14285,#9064,.T.);
#17957=EDGE_CURVE('',#14296,#14295,#9065,.T.);
#17958=EDGE_CURVE('',#14294,#14296,#9066,.T.);
#17959=EDGE_CURVE('',#14259,#14295,#9067,.T.);
#17960=EDGE_CURVE('',#14292,#14297,#9068,.T.);
#17961=EDGE_CURVE('',#14297,#14298,#9069,.T.);
#17962=EDGE_CURVE('',#14258,#14298,#9070,.T.);
#17963=EDGE_CURVE('',#14299,#14299,#2728,.T.);
#17964=EDGE_CURVE('',#14300,#14300,#2729,.T.);
#17965=EDGE_CURVE('',#14301,#14302,#9071,.T.);
#17966=EDGE_CURVE('',#14302,#14303,#9072,.T.);
#17967=EDGE_CURVE('',#14303,#14304,#9073,.T.);
#17968=EDGE_CURVE('',#14304,#14301,#9074,.T.);
#17969=EDGE_CURVE('',#14305,#14305,#2730,.T.);
#17970=EDGE_CURVE('',#14306,#14306,#2731,.T.);
#17971=EDGE_CURVE('',#14307,#14307,#2732,.T.);
#17972=EDGE_CURVE('',#14307,#14299,#9075,.T.);
#17973=EDGE_CURVE('',#14307,#14308,#9076,.T.);
#17974=EDGE_CURVE('',#14309,#14308,#2733,.T.);
#17975=EDGE_CURVE('',#14308,#14309,#2734,.T.);
#17976=EDGE_CURVE('',#14310,#14310,#2735,.T.);
#17977=EDGE_CURVE('',#14310,#14306,#9077,.T.);
#17978=EDGE_CURVE('',#14310,#14311,#9078,.T.);
#17979=EDGE_CURVE('',#14312,#14311,#2736,.T.);
#17980=EDGE_CURVE('',#14311,#14312,#2737,.T.);
#17981=EDGE_CURVE('',#14313,#14313,#2738,.T.);
#17982=EDGE_CURVE('',#14313,#14300,#9079,.T.);
#17983=EDGE_CURVE('',#14313,#14314,#9080,.T.);
#17984=EDGE_CURVE('',#14315,#14314,#2739,.T.);
#17985=EDGE_CURVE('',#14314,#14315,#2740,.T.);
#17986=EDGE_CURVE('',#14316,#14316,#2741,.T.);
#17987=EDGE_CURVE('',#14316,#14305,#9081,.T.);
#17988=EDGE_CURVE('',#14316,#14317,#9082,.T.);
#17989=EDGE_CURVE('',#14318,#14317,#2742,.T.);
#17990=EDGE_CURVE('',#14317,#14318,#2743,.T.);
#17991=EDGE_CURVE('',#14309,#14231,#9083,.T.);
#17992=EDGE_CURVE('',#14312,#14224,#9084,.T.);
#17993=EDGE_CURVE('',#14315,#14230,#9085,.T.);
#17994=EDGE_CURVE('',#14318,#14225,#9086,.T.);
#17995=EDGE_CURVE('',#14214,#14296,#9087,.T.);
#17996=EDGE_CURVE('',#14319,#14297,#9088,.T.);
#17997=EDGE_CURVE('',#14320,#14319,#9089,.T.);
#17998=EDGE_CURVE('',#14298,#14320,#9090,.T.);
#17999=EDGE_CURVE('',#14217,#14320,#9091,.T.);
#18000=EDGE_CURVE('',#14247,#14319,#9092,.T.);
#18001=EDGE_CURVE('',#14321,#14293,#9093,.T.);
#18002=EDGE_CURVE('',#14223,#14321,#9094,.T.);
#18003=EDGE_CURVE('',#14234,#14321,#9095,.T.);
#18004=EDGE_CURVE('',#14253,#14235,#9096,.T.);
#18005=EDGE_CURVE('',#14228,#14304,#9097,.T.);
#18006=EDGE_CURVE('',#14303,#14229,#9098,.T.);
#18007=EDGE_CURVE('',#14226,#14302,#9099,.T.);
#18008=EDGE_CURVE('',#14227,#14301,#9100,.T.);
#23838=ORIENTED_EDGE('',*,*,#17821,.T.);
#23839=ORIENTED_EDGE('',*,*,#17822,.T.);
#23840=ORIENTED_EDGE('',*,*,#17823,.T.);
#23841=ORIENTED_EDGE('',*,*,#17824,.T.);
#23842=ORIENTED_EDGE('',*,*,#17822,.F.);
#23843=ORIENTED_EDGE('',*,*,#17825,.T.);
#23844=ORIENTED_EDGE('',*,*,#17826,.T.);
#23845=ORIENTED_EDGE('',*,*,#17827,.F.);
#23846=ORIENTED_EDGE('',*,*,#17828,.T.);
#23847=ORIENTED_EDGE('',*,*,#17829,.T.);
#23848=ORIENTED_EDGE('',*,*,#17830,.F.);
#23849=ORIENTED_EDGE('',*,*,#17831,.T.);
#23850=ORIENTED_EDGE('',*,*,#17832,.T.);
#23851=ORIENTED_EDGE('',*,*,#17833,.F.);
#23852=ORIENTED_EDGE('',*,*,#17834,.T.);
#23853=ORIENTED_EDGE('',*,*,#17835,.T.);
#23854=ORIENTED_EDGE('',*,*,#17836,.F.);
#23855=ORIENTED_EDGE('',*,*,#17837,.F.);
#23856=ORIENTED_EDGE('',*,*,#17838,.T.);
#23857=ORIENTED_EDGE('',*,*,#17839,.T.);
#23858=ORIENTED_EDGE('',*,*,#17840,.T.);
#23859=ORIENTED_EDGE('',*,*,#17841,.T.);
#23860=ORIENTED_EDGE('',*,*,#17842,.F.);
#23861=ORIENTED_EDGE('',*,*,#17843,.F.);
#23862=ORIENTED_EDGE('',*,*,#17844,.T.);
#23863=ORIENTED_EDGE('',*,*,#17845,.T.);
#23864=ORIENTED_EDGE('',*,*,#17846,.T.);
#23865=ORIENTED_EDGE('',*,*,#17833,.T.);
#23866=ORIENTED_EDGE('',*,*,#17847,.F.);
#23867=ORIENTED_EDGE('',*,*,#17845,.F.);
#23868=ORIENTED_EDGE('',*,*,#17848,.T.);
#23869=ORIENTED_EDGE('',*,*,#17849,.T.);
#23870=ORIENTED_EDGE('',*,*,#17850,.F.);
#23871=ORIENTED_EDGE('',*,*,#17851,.F.);
#23872=ORIENTED_EDGE('',*,*,#17852,.F.);
#23873=ORIENTED_EDGE('',*,*,#17853,.F.);
#23874=ORIENTED_EDGE('',*,*,#17854,.F.);
#23875=ORIENTED_EDGE('',*,*,#17855,.F.);
#23876=ORIENTED_EDGE('',*,*,#17856,.F.);
#23877=ORIENTED_EDGE('',*,*,#17857,.F.);
#23878=ORIENTED_EDGE('',*,*,#17858,.F.);
#23879=ORIENTED_EDGE('',*,*,#17859,.T.);
#23880=ORIENTED_EDGE('',*,*,#17860,.F.);
#23881=ORIENTED_EDGE('',*,*,#17830,.T.);
#23882=ORIENTED_EDGE('',*,*,#17861,.F.);
#23883=ORIENTED_EDGE('',*,*,#17862,.T.);
#23884=ORIENTED_EDGE('',*,*,#17863,.T.);
#23885=ORIENTED_EDGE('',*,*,#17864,.T.);
#23886=ORIENTED_EDGE('',*,*,#17865,.F.);
#23887=ORIENTED_EDGE('',*,*,#17866,.T.);
#23888=ORIENTED_EDGE('',*,*,#17862,.F.);
#23889=ORIENTED_EDGE('',*,*,#17867,.F.);
#23890=ORIENTED_EDGE('',*,*,#17864,.F.);
#23891=ORIENTED_EDGE('',*,*,#17868,.T.);
#23892=ORIENTED_EDGE('',*,*,#17860,.T.);
#23893=ORIENTED_EDGE('',*,*,#17869,.T.);
#23894=ORIENTED_EDGE('',*,*,#17870,.T.);
#23895=ORIENTED_EDGE('',*,*,#17871,.F.);
#23896=ORIENTED_EDGE('',*,*,#17831,.F.);
#23897=ORIENTED_EDGE('',*,*,#17867,.T.);
#23898=ORIENTED_EDGE('',*,*,#17872,.T.);
#23899=ORIENTED_EDGE('',*,*,#17873,.F.);
#23900=ORIENTED_EDGE('',*,*,#17850,.T.);
#23901=ORIENTED_EDGE('',*,*,#17874,.T.);
#23902=ORIENTED_EDGE('',*,*,#17869,.F.);
#23903=ORIENTED_EDGE('',*,*,#17868,.F.);
#23904=ORIENTED_EDGE('',*,*,#17863,.F.);
#23905=ORIENTED_EDGE('',*,*,#17866,.F.);
#23906=ORIENTED_EDGE('',*,*,#17875,.F.);
#23907=ORIENTED_EDGE('',*,*,#17876,.F.);
#23908=ORIENTED_EDGE('',*,*,#17877,.F.);
#23909=ORIENTED_EDGE('',*,*,#17878,.F.);
#23910=ORIENTED_EDGE('',*,*,#17872,.F.);
#23911=ORIENTED_EDGE('',*,*,#17879,.T.);
#23912=ORIENTED_EDGE('',*,*,#17827,.T.);
#23913=ORIENTED_EDGE('',*,*,#17880,.T.);
#23914=ORIENTED_EDGE('',*,*,#17881,.T.);
#23915=ORIENTED_EDGE('',*,*,#17882,.F.);
#23916=ORIENTED_EDGE('',*,*,#17883,.F.);
#23917=ORIENTED_EDGE('',*,*,#17884,.F.);
#23918=ORIENTED_EDGE('',*,*,#17885,.F.);
#23919=ORIENTED_EDGE('',*,*,#17886,.F.);
#23920=ORIENTED_EDGE('',*,*,#17887,.F.);
#23921=ORIENTED_EDGE('',*,*,#17888,.F.);
#23922=ORIENTED_EDGE('',*,*,#17889,.F.);
#23923=ORIENTED_EDGE('',*,*,#17890,.F.);
#23924=ORIENTED_EDGE('',*,*,#17891,.F.);
#23925=ORIENTED_EDGE('',*,*,#17892,.F.);
#23926=ORIENTED_EDGE('',*,*,#17893,.F.);
#23927=ORIENTED_EDGE('',*,*,#17894,.F.);
#23928=ORIENTED_EDGE('',*,*,#17895,.F.);
#23929=ORIENTED_EDGE('',*,*,#17896,.F.);
#23930=ORIENTED_EDGE('',*,*,#17897,.F.);
#23931=ORIENTED_EDGE('',*,*,#17898,.F.);
#23932=ORIENTED_EDGE('',*,*,#17899,.F.);
#23933=ORIENTED_EDGE('',*,*,#17900,.T.);
#23934=ORIENTED_EDGE('',*,*,#17901,.F.);
#23935=ORIENTED_EDGE('',*,*,#17902,.F.);
#23936=ORIENTED_EDGE('',*,*,#17903,.F.);
#23937=ORIENTED_EDGE('',*,*,#17904,.F.);
#23938=ORIENTED_EDGE('',*,*,#17905,.F.);
#23939=ORIENTED_EDGE('',*,*,#17855,.T.);
#23940=ORIENTED_EDGE('',*,*,#17906,.F.);
#23941=ORIENTED_EDGE('',*,*,#17907,.F.);
#23942=ORIENTED_EDGE('',*,*,#17908,.F.);
#23943=ORIENTED_EDGE('',*,*,#17909,.F.);
#23944=ORIENTED_EDGE('',*,*,#17910,.F.);
#23945=ORIENTED_EDGE('',*,*,#17911,.F.);
#23946=ORIENTED_EDGE('',*,*,#17912,.F.);
#23947=ORIENTED_EDGE('',*,*,#17908,.T.);
#23948=ORIENTED_EDGE('',*,*,#17913,.T.);
#23949=ORIENTED_EDGE('',*,*,#17911,.T.);
#23950=ORIENTED_EDGE('',*,*,#17914,.T.);
#23951=ORIENTED_EDGE('',*,*,#17915,.T.);
#23952=ORIENTED_EDGE('',*,*,#17916,.T.);
#23953=ORIENTED_EDGE('',*,*,#17912,.T.);
#23954=ORIENTED_EDGE('',*,*,#17917,.T.);
#23955=ORIENTED_EDGE('',*,*,#17918,.F.);
#23956=ORIENTED_EDGE('',*,*,#17919,.F.);
#23957=ORIENTED_EDGE('',*,*,#17920,.F.);
#23958=ORIENTED_EDGE('',*,*,#17905,.T.);
#23959=ORIENTED_EDGE('',*,*,#17921,.T.);
#23960=ORIENTED_EDGE('',*,*,#17919,.T.);
#23961=ORIENTED_EDGE('',*,*,#17856,.T.);
#23962=ORIENTED_EDGE('',*,*,#17920,.T.);
#23963=ORIENTED_EDGE('',*,*,#17922,.T.);
#23964=ORIENTED_EDGE('',*,*,#17909,.T.);
#23965=ORIENTED_EDGE('',*,*,#17923,.T.);
#23966=ORIENTED_EDGE('',*,*,#17924,.F.);
#23967=ORIENTED_EDGE('',*,*,#17925,.F.);
#23968=ORIENTED_EDGE('',*,*,#17926,.F.);
#23969=ORIENTED_EDGE('',*,*,#17927,.T.);
#23970=ORIENTED_EDGE('',*,*,#17858,.T.);
#23971=ORIENTED_EDGE('',*,*,#17925,.T.);
#23972=ORIENTED_EDGE('',*,*,#17928,.T.);
#23973=ORIENTED_EDGE('',*,*,#17918,.T.);
#23974=ORIENTED_EDGE('',*,*,#17929,.T.);
#23975=ORIENTED_EDGE('',*,*,#17926,.T.);
#23976=ORIENTED_EDGE('',*,*,#17857,.T.);
#23977=ORIENTED_EDGE('',*,*,#17924,.T.);
#23978=ORIENTED_EDGE('',*,*,#17930,.T.);
#23979=ORIENTED_EDGE('',*,*,#17910,.T.);
#23980=ORIENTED_EDGE('',*,*,#17931,.T.);
#23981=ORIENTED_EDGE('',*,*,#17901,.T.);
#23982=ORIENTED_EDGE('',*,*,#17932,.T.);
#23983=ORIENTED_EDGE('',*,*,#17907,.T.);
#23984=ORIENTED_EDGE('',*,*,#17933,.T.);
#23985=ORIENTED_EDGE('',*,*,#17898,.T.);
#23986=ORIENTED_EDGE('',*,*,#17934,.T.);
#23987=ORIENTED_EDGE('',*,*,#17906,.T.);
#23988=ORIENTED_EDGE('',*,*,#17854,.T.);
#23989=ORIENTED_EDGE('',*,*,#17904,.T.);
#23990=ORIENTED_EDGE('',*,*,#17935,.T.);
#23991=ORIENTED_EDGE('',*,*,#17902,.T.);
#23992=ORIENTED_EDGE('',*,*,#17936,.T.);
#23993=ORIENTED_EDGE('',*,*,#17895,.T.);
#23994=ORIENTED_EDGE('',*,*,#17937,.T.);
#23995=ORIENTED_EDGE('',*,*,#17903,.T.);
#23996=ORIENTED_EDGE('',*,*,#17938,.T.);
#23997=ORIENTED_EDGE('',*,*,#17892,.T.);
#23998=ORIENTED_EDGE('',*,*,#17939,.T.);
#23999=ORIENTED_EDGE('',*,*,#17899,.T.);
#24000=ORIENTED_EDGE('',*,*,#17853,.T.);
#24001=ORIENTED_EDGE('',*,*,#17897,.T.);
#24002=ORIENTED_EDGE('',*,*,#17940,.T.);
#24003=ORIENTED_EDGE('',*,*,#17896,.T.);
#24004=ORIENTED_EDGE('',*,*,#17941,.T.);
#24005=ORIENTED_EDGE('',*,*,#17889,.T.);
#24006=ORIENTED_EDGE('',*,*,#17942,.T.);
#24007=ORIENTED_EDGE('',*,*,#17894,.T.);
#24008=ORIENTED_EDGE('',*,*,#17943,.T.);
#24009=ORIENTED_EDGE('',*,*,#17886,.T.);
#24010=ORIENTED_EDGE('',*,*,#17944,.T.);
#24011=ORIENTED_EDGE('',*,*,#17893,.T.);
#24012=ORIENTED_EDGE('',*,*,#17852,.T.);
#24013=ORIENTED_EDGE('',*,*,#17891,.T.);
#24014=ORIENTED_EDGE('',*,*,#17945,.T.);
#24015=ORIENTED_EDGE('',*,*,#17890,.T.);
#24016=ORIENTED_EDGE('',*,*,#17946,.T.);
#24017=ORIENTED_EDGE('',*,*,#17883,.T.);
#24018=ORIENTED_EDGE('',*,*,#17947,.T.);
#24019=ORIENTED_EDGE('',*,*,#17888,.T.);
#24020=ORIENTED_EDGE('',*,*,#17948,.T.);
#24021=ORIENTED_EDGE('',*,*,#17873,.T.);
#24022=ORIENTED_EDGE('',*,*,#17878,.T.);
#24023=ORIENTED_EDGE('',*,*,#17887,.T.);
#24024=ORIENTED_EDGE('',*,*,#17851,.T.);
#24025=ORIENTED_EDGE('',*,*,#17885,.T.);
#24026=ORIENTED_EDGE('',*,*,#17877,.T.);
#24027=ORIENTED_EDGE('',*,*,#17884,.T.);
#24028=ORIENTED_EDGE('',*,*,#17949,.T.);
#24029=ORIENTED_EDGE('',*,*,#17950,.T.);
#24030=ORIENTED_EDGE('',*,*,#17951,.T.);
#24031=ORIENTED_EDGE('',*,*,#17882,.T.);
#24032=ORIENTED_EDGE('',*,*,#17876,.T.);
#24033=ORIENTED_EDGE('',*,*,#17952,.T.);
#24034=ORIENTED_EDGE('',*,*,#17953,.T.);
#24035=ORIENTED_EDGE('',*,*,#17928,.F.);
#24036=ORIENTED_EDGE('',*,*,#17931,.F.);
#24037=ORIENTED_EDGE('',*,*,#17916,.F.);
#24038=ORIENTED_EDGE('',*,*,#17954,.T.);
#24039=ORIENTED_EDGE('',*,*,#17955,.F.);
#24040=ORIENTED_EDGE('',*,*,#17824,.F.);
#24041=ORIENTED_EDGE('',*,*,#17915,.F.);
#24042=ORIENTED_EDGE('',*,*,#17956,.F.);
#24043=ORIENTED_EDGE('',*,*,#17957,.F.);
#24044=ORIENTED_EDGE('',*,*,#17958,.F.);
#24045=ORIENTED_EDGE('',*,*,#17954,.F.);
#24046=ORIENTED_EDGE('',*,*,#17959,.T.);
#24047=ORIENTED_EDGE('',*,*,#17956,.T.);
#24048=ORIENTED_EDGE('',*,*,#17917,.F.);
#24049=ORIENTED_EDGE('',*,*,#17913,.F.);
#24050=ORIENTED_EDGE('',*,*,#17932,.F.);
#24051=ORIENTED_EDGE('',*,*,#17900,.F.);
#24052=ORIENTED_EDGE('',*,*,#17937,.F.);
#24053=ORIENTED_EDGE('',*,*,#17942,.F.);
#24054=ORIENTED_EDGE('',*,*,#17947,.F.);
#24055=ORIENTED_EDGE('',*,*,#17951,.F.);
#24056=ORIENTED_EDGE('',*,*,#17960,.T.);
#24057=ORIENTED_EDGE('',*,*,#17961,.T.);
#24058=ORIENTED_EDGE('',*,*,#17962,.F.);
#24059=ORIENTED_EDGE('',*,*,#17881,.F.);
#24060=ORIENTED_EDGE('',*,*,#17914,.F.);
#24061=ORIENTED_EDGE('',*,*,#17930,.F.);
#24062=ORIENTED_EDGE('',*,*,#17929,.F.);
#24063=ORIENTED_EDGE('',*,*,#17923,.F.);
#24064=ORIENTED_EDGE('',*,*,#17963,.F.);
#24065=ORIENTED_EDGE('',*,*,#17964,.F.);
#24066=ORIENTED_EDGE('',*,*,#17965,.T.);
#24067=ORIENTED_EDGE('',*,*,#17966,.T.);
#24068=ORIENTED_EDGE('',*,*,#17967,.T.);
#24069=ORIENTED_EDGE('',*,*,#17968,.T.);
#24070=ORIENTED_EDGE('',*,*,#17969,.F.);
#24071=ORIENTED_EDGE('',*,*,#17970,.F.);
#24072=ORIENTED_EDGE('',*,*,#17921,.F.);
#24073=ORIENTED_EDGE('',*,*,#17936,.F.);
#24074=ORIENTED_EDGE('',*,*,#17933,.F.);
#24075=ORIENTED_EDGE('',*,*,#17922,.F.);
#24076=ORIENTED_EDGE('',*,*,#17934,.F.);
#24077=ORIENTED_EDGE('',*,*,#17941,.F.);
#24078=ORIENTED_EDGE('',*,*,#17938,.F.);
#24079=ORIENTED_EDGE('',*,*,#17935,.F.);
#24080=ORIENTED_EDGE('',*,*,#17939,.F.);
#24081=ORIENTED_EDGE('',*,*,#17946,.F.);
#24082=ORIENTED_EDGE('',*,*,#17943,.F.);
#24083=ORIENTED_EDGE('',*,*,#17940,.F.);
#24084=ORIENTED_EDGE('',*,*,#17944,.F.);
#24085=ORIENTED_EDGE('',*,*,#17949,.F.);
#24086=ORIENTED_EDGE('',*,*,#17948,.F.);
#24087=ORIENTED_EDGE('',*,*,#17945,.F.);
#24088=ORIENTED_EDGE('',*,*,#17971,.T.);
#24089=ORIENTED_EDGE('',*,*,#17972,.T.);
#24090=ORIENTED_EDGE('',*,*,#17963,.T.);
#24091=ORIENTED_EDGE('',*,*,#17972,.F.);
#24092=ORIENTED_EDGE('',*,*,#17971,.F.);
#24093=ORIENTED_EDGE('',*,*,#17973,.T.);
#24094=ORIENTED_EDGE('',*,*,#17974,.F.);
#24095=ORIENTED_EDGE('',*,*,#17975,.F.);
#24096=ORIENTED_EDGE('',*,*,#17973,.F.);
#24097=ORIENTED_EDGE('',*,*,#17976,.T.);
#24098=ORIENTED_EDGE('',*,*,#17977,.T.);
#24099=ORIENTED_EDGE('',*,*,#17970,.T.);
#24100=ORIENTED_EDGE('',*,*,#17977,.F.);
#24101=ORIENTED_EDGE('',*,*,#17976,.F.);
#24102=ORIENTED_EDGE('',*,*,#17978,.T.);
#24103=ORIENTED_EDGE('',*,*,#17979,.F.);
#24104=ORIENTED_EDGE('',*,*,#17980,.F.);
#24105=ORIENTED_EDGE('',*,*,#17978,.F.);
#24106=ORIENTED_EDGE('',*,*,#17981,.T.);
#24107=ORIENTED_EDGE('',*,*,#17982,.T.);
#24108=ORIENTED_EDGE('',*,*,#17964,.T.);
#24109=ORIENTED_EDGE('',*,*,#17982,.F.);
#24110=ORIENTED_EDGE('',*,*,#17981,.F.);
#24111=ORIENTED_EDGE('',*,*,#17983,.T.);
#24112=ORIENTED_EDGE('',*,*,#17984,.F.);
#24113=ORIENTED_EDGE('',*,*,#17985,.F.);
#24114=ORIENTED_EDGE('',*,*,#17983,.F.);
#24115=ORIENTED_EDGE('',*,*,#17986,.T.);
#24116=ORIENTED_EDGE('',*,*,#17987,.T.);
#24117=ORIENTED_EDGE('',*,*,#17969,.T.);
#24118=ORIENTED_EDGE('',*,*,#17987,.F.);
#24119=ORIENTED_EDGE('',*,*,#17986,.F.);
#24120=ORIENTED_EDGE('',*,*,#17988,.T.);
#24121=ORIENTED_EDGE('',*,*,#17989,.F.);
#24122=ORIENTED_EDGE('',*,*,#17990,.F.);
#24123=ORIENTED_EDGE('',*,*,#17988,.F.);
#24124=ORIENTED_EDGE('',*,*,#17974,.T.);
#24125=ORIENTED_EDGE('',*,*,#17975,.T.);
#24126=ORIENTED_EDGE('',*,*,#17991,.T.);
#24127=ORIENTED_EDGE('',*,*,#17843,.T.);
#24128=ORIENTED_EDGE('',*,*,#17991,.F.);
#24129=ORIENTED_EDGE('',*,*,#17979,.T.);
#24130=ORIENTED_EDGE('',*,*,#17980,.T.);
#24131=ORIENTED_EDGE('',*,*,#17992,.T.);
#24132=ORIENTED_EDGE('',*,*,#17836,.T.);
#24133=ORIENTED_EDGE('',*,*,#17992,.F.);
#24134=ORIENTED_EDGE('',*,*,#17984,.T.);
#24135=ORIENTED_EDGE('',*,*,#17985,.T.);
#24136=ORIENTED_EDGE('',*,*,#17993,.T.);
#24137=ORIENTED_EDGE('',*,*,#17842,.T.);
#24138=ORIENTED_EDGE('',*,*,#17993,.F.);
#24139=ORIENTED_EDGE('',*,*,#17989,.T.);
#24140=ORIENTED_EDGE('',*,*,#17990,.T.);
#24141=ORIENTED_EDGE('',*,*,#17994,.T.);
#24142=ORIENTED_EDGE('',*,*,#17837,.T.);
#24143=ORIENTED_EDGE('',*,*,#17994,.F.);
#24144=ORIENTED_EDGE('',*,*,#17957,.T.);
#24145=ORIENTED_EDGE('',*,*,#17959,.F.);
#24146=ORIENTED_EDGE('',*,*,#17880,.F.);
#24147=ORIENTED_EDGE('',*,*,#17826,.F.);
#24148=ORIENTED_EDGE('',*,*,#17995,.T.);
#24149=ORIENTED_EDGE('',*,*,#17958,.T.);
#24150=ORIENTED_EDGE('',*,*,#17995,.F.);
#24151=ORIENTED_EDGE('',*,*,#17825,.F.);
#24152=ORIENTED_EDGE('',*,*,#17821,.F.);
#24153=ORIENTED_EDGE('',*,*,#17955,.T.);
#24154=ORIENTED_EDGE('',*,*,#17961,.F.);
#24155=ORIENTED_EDGE('',*,*,#17996,.F.);
#24156=ORIENTED_EDGE('',*,*,#17997,.F.);
#24157=ORIENTED_EDGE('',*,*,#17998,.F.);
#24158=ORIENTED_EDGE('',*,*,#17998,.T.);
#24159=ORIENTED_EDGE('',*,*,#17999,.F.);
#24160=ORIENTED_EDGE('',*,*,#17828,.F.);
#24161=ORIENTED_EDGE('',*,*,#17879,.F.);
#24162=ORIENTED_EDGE('',*,*,#17962,.T.);
#24163=ORIENTED_EDGE('',*,*,#17865,.T.);
#24164=ORIENTED_EDGE('',*,*,#18000,.T.);
#24165=ORIENTED_EDGE('',*,*,#17996,.T.);
#24166=ORIENTED_EDGE('',*,*,#17960,.F.);
#24167=ORIENTED_EDGE('',*,*,#17950,.F.);
#24168=ORIENTED_EDGE('',*,*,#17875,.T.);
#24169=ORIENTED_EDGE('',*,*,#17861,.T.);
#24170=ORIENTED_EDGE('',*,*,#17829,.F.);
#24171=ORIENTED_EDGE('',*,*,#17999,.T.);
#24172=ORIENTED_EDGE('',*,*,#17997,.T.);
#24173=ORIENTED_EDGE('',*,*,#18000,.F.);
#24174=ORIENTED_EDGE('',*,*,#18001,.T.);
#24175=ORIENTED_EDGE('',*,*,#17952,.F.);
#24176=ORIENTED_EDGE('',*,*,#17823,.F.);
#24177=ORIENTED_EDGE('',*,*,#17835,.F.);
#24178=ORIENTED_EDGE('',*,*,#18002,.T.);
#24179=ORIENTED_EDGE('',*,*,#18003,.T.);
#24180=ORIENTED_EDGE('',*,*,#18002,.F.);
#24181=ORIENTED_EDGE('',*,*,#17834,.F.);
#24182=ORIENTED_EDGE('',*,*,#17846,.F.);
#24183=ORIENTED_EDGE('',*,*,#17847,.T.);
#24184=ORIENTED_EDGE('',*,*,#17927,.F.);
#24185=ORIENTED_EDGE('',*,*,#17953,.F.);
#24186=ORIENTED_EDGE('',*,*,#18001,.F.);
#24187=ORIENTED_EDGE('',*,*,#18003,.F.);
#24188=ORIENTED_EDGE('',*,*,#17859,.F.);
#24189=ORIENTED_EDGE('',*,*,#17849,.F.);
#24190=ORIENTED_EDGE('',*,*,#18004,.F.);
#24191=ORIENTED_EDGE('',*,*,#17870,.F.);
#24192=ORIENTED_EDGE('',*,*,#17874,.F.);
#24193=ORIENTED_EDGE('',*,*,#18004,.T.);
#24194=ORIENTED_EDGE('',*,*,#17848,.F.);
#24195=ORIENTED_EDGE('',*,*,#17844,.F.);
#24196=ORIENTED_EDGE('',*,*,#17832,.F.);
#24197=ORIENTED_EDGE('',*,*,#17871,.T.);
#24198=ORIENTED_EDGE('',*,*,#17840,.F.);
#24199=ORIENTED_EDGE('',*,*,#18005,.T.);
#24200=ORIENTED_EDGE('',*,*,#17967,.F.);
#24201=ORIENTED_EDGE('',*,*,#18006,.T.);
#24202=ORIENTED_EDGE('',*,*,#17841,.F.);
#24203=ORIENTED_EDGE('',*,*,#18006,.F.);
#24204=ORIENTED_EDGE('',*,*,#17966,.F.);
#24205=ORIENTED_EDGE('',*,*,#18007,.F.);
#24206=ORIENTED_EDGE('',*,*,#17838,.F.);
#24207=ORIENTED_EDGE('',*,*,#18007,.T.);
#24208=ORIENTED_EDGE('',*,*,#17965,.F.);
#24209=ORIENTED_EDGE('',*,*,#18008,.F.);
#24210=ORIENTED_EDGE('',*,*,#17839,.F.);
#24211=ORIENTED_EDGE('',*,*,#18008,.T.);
#24212=ORIENTED_EDGE('',*,*,#17968,.F.);
#24213=ORIENTED_EDGE('',*,*,#18005,.F.);
#31400=PLANE('',#35044);
#31401=PLANE('',#35052);
#31402=PLANE('',#35061);
#31403=PLANE('',#35062);
#31404=PLANE('',#35064);
#31405=PLANE('',#35140);
#31406=PLANE('',#35141);
#31407=PLANE('',#35142);
#31408=PLANE('',#35143);
#31409=PLANE('',#35148);
#31410=PLANE('',#35149);
#31411=PLANE('',#35150);
#31412=PLANE('',#35151);
#31413=PLANE('',#35176);
#31414=PLANE('',#35177);
#31415=PLANE('',#35178);
#31416=PLANE('',#35179);
#31417=PLANE('',#35180);
#31418=PLANE('',#35181);
#31419=PLANE('',#35182);
#31420=PLANE('',#35183);
#31421=PLANE('',#35184);
#31422=PLANE('',#35185);
#31423=PLANE('',#35186);
#31424=PLANE('',#35187);
#31425=PLANE('',#35188);
#31426=PLANE('',#35189);
#31427=PLANE('',#35190);
#32409=ADVANCED_FACE('',(#4728),#1163,.T.);
#32410=ADVANCED_FACE('',(#4729,#1968,#1969,#1970,#1971,#1972),#31400,.T.);
#32411=ADVANCED_FACE('',(#4730),#1164,.T.);
#32412=ADVANCED_FACE('',(#4731),#31401,.T.);
#32413=ADVANCED_FACE('',(#4732),#1165,.F.);
#32414=ADVANCED_FACE('',(#4733),#474,.T.);
#32415=ADVANCED_FACE('',(#4734),#475,.T.);
#32416=ADVANCED_FACE('',(#4735),#31402,.T.);
#32417=ADVANCED_FACE('',(#4736),#31403,.T.);
#32418=ADVANCED_FACE('',(#4737),#31404,.T.);
#32419=ADVANCED_FACE('',(#4738),#1166,.T.);
#32420=ADVANCED_FACE('',(#4739),#733,.T.);
#32421=ADVANCED_FACE('',(#4740),#734,.T.);
#32422=ADVANCED_FACE('',(#4741),#735,.T.);
#32423=ADVANCED_FACE('',(#4742),#736,.T.);
#32424=ADVANCED_FACE('',(#4743),#737,.T.);
#32425=ADVANCED_FACE('',(#4744),#738,.T.);
#32426=ADVANCED_FACE('',(#4745),#896,.T.);
#32427=ADVANCED_FACE('',(#4746),#897,.T.);
#32428=ADVANCED_FACE('',(#4747),#739,.T.);
#32429=ADVANCED_FACE('',(#4748),#740,.T.);
#32430=ADVANCED_FACE('',(#4749),#1167,.T.);
#32431=ADVANCED_FACE('',(#4750),#1168,.T.);
#32432=ADVANCED_FACE('',(#4751),#741,.T.);
#32433=ADVANCED_FACE('',(#4752),#1169,.T.);
#32434=ADVANCED_FACE('',(#4753),#1170,.T.);
#32435=ADVANCED_FACE('',(#4754),#742,.T.);
#32436=ADVANCED_FACE('',(#4755),#1171,.T.);
#32437=ADVANCED_FACE('',(#4756),#1172,.T.);
#32438=ADVANCED_FACE('',(#4757),#1173,.T.);
#32439=ADVANCED_FACE('',(#4758),#1174,.T.);
#32440=ADVANCED_FACE('',(#4759),#1175,.T.);
#32441=ADVANCED_FACE('',(#4760),#1176,.F.);
#32442=ADVANCED_FACE('',(#4761),#1177,.T.);
#32443=ADVANCED_FACE('',(#4762),#1178,.T.);
#32444=ADVANCED_FACE('',(#4763),#1179,.T.);
#32445=ADVANCED_FACE('',(#4764),#1180,.T.);
#32446=ADVANCED_FACE('',(#4765),#1181,.T.);
#32447=ADVANCED_FACE('',(#4766),#1182,.T.);
#32448=ADVANCED_FACE('',(#4767),#1183,.T.);
#32449=ADVANCED_FACE('',(#4768),#1184,.T.);
#32450=ADVANCED_FACE('',(#4769),#1185,.T.);
#32451=ADVANCED_FACE('',(#4770),#1186,.T.);
#32452=ADVANCED_FACE('',(#4771),#31405,.T.);
#32453=ADVANCED_FACE('',(#4772),#31406,.T.);
#32454=ADVANCED_FACE('',(#4773),#31407,.T.);
#32455=ADVANCED_FACE('',(#4774,#1973,#1974,#1975,#1976,#1977),#31408,.T.);
#32456=ADVANCED_FACE('',(#4775),#31409,.T.);
#32457=ADVANCED_FACE('',(#4776),#31410,.T.);
#32458=ADVANCED_FACE('',(#4777),#31411,.T.);
#32459=ADVANCED_FACE('',(#4778),#31412,.T.);
#32460=ADVANCED_FACE('',(#4779),#583,.F.);
#32461=ADVANCED_FACE('',(#4780),#1187,.F.);
#32462=ADVANCED_FACE('',(#4781),#584,.F.);
#32463=ADVANCED_FACE('',(#4782),#1188,.F.);
#32464=ADVANCED_FACE('',(#4783),#585,.F.);
#32465=ADVANCED_FACE('',(#4784),#1189,.F.);
#32466=ADVANCED_FACE('',(#4785),#586,.F.);
#32467=ADVANCED_FACE('',(#4786),#1190,.F.);
#32468=ADVANCED_FACE('',(#4787),#587,.F.);
#32469=ADVANCED_FACE('',(#4788),#588,.F.);
#32470=ADVANCED_FACE('',(#4789),#589,.F.);
#32471=ADVANCED_FACE('',(#4790),#590,.F.);
#32472=ADVANCED_FACE('',(#4791),#31413,.T.);
#32473=ADVANCED_FACE('',(#4792),#31414,.T.);
#32474=ADVANCED_FACE('',(#4793),#31415,.T.);
#32475=ADVANCED_FACE('',(#4794),#31416,.T.);
#32476=ADVANCED_FACE('',(#4795),#31417,.T.);
#32477=ADVANCED_FACE('',(#4796),#31418,.T.);
#32478=ADVANCED_FACE('',(#4797),#31419,.T.);
#32479=ADVANCED_FACE('',(#4798),#31420,.T.);
#32480=ADVANCED_FACE('',(#4799),#31421,.T.);
#32481=ADVANCED_FACE('',(#4800),#31422,.T.);
#32482=ADVANCED_FACE('',(#4801),#31423,.T.);
#32483=ADVANCED_FACE('',(#4802),#31424,.F.);
#32484=ADVANCED_FACE('',(#4803),#31425,.F.);
#32485=ADVANCED_FACE('',(#4804),#31426,.F.);
#32486=ADVANCED_FACE('',(#4805),#31427,.F.);
#33800=CLOSED_SHELL('',(#32409,#32410,#32411,#32412,#32413,#32414,#32415,
#32416,#32417,#32418,#32419,#32420,#32421,#32422,#32423,#32424,#32425,#32426,
#32427,#32428,#32429,#32430,#32431,#32432,#32433,#32434,#32435,#32436,#32437,
#32438,#32439,#32440,#32441,#32442,#32443,#32444,#32445,#32446,#32447,#32448,
#32449,#32450,#32451,#32452,#32453,#32454,#32455,#32456,#32457,#32458,#32459,
#32460,#32461,#32462,#32463,#32464,#32465,#32466,#32467,#32468,#32469,#32470,
#32471,#32472,#32473,#32474,#32475,#32476,#32477,#32478,#32479,#32480,#32481,
#32482,#32483,#32484,#32485,#32486));
#35040=AXIS2_PLACEMENT_3D('',#53354,#40665,#40666);
#35041=AXIS2_PLACEMENT_3D('',#53355,#40667,#40668);
#35042=AXIS2_PLACEMENT_3D('',#53358,#40669,#40670);
#35043=AXIS2_PLACEMENT_3D('',#53362,#40672,#40673);
#35044=AXIS2_PLACEMENT_3D('',#53364,#40675,#40676);
#35045=AXIS2_PLACEMENT_3D('',#53387,#40688,#40689);
#35046=AXIS2_PLACEMENT_3D('',#53389,#40690,#40691);
#35047=AXIS2_PLACEMENT_3D('',#53399,#40696,#40697);
#35048=AXIS2_PLACEMENT_3D('',#53401,#40698,#40699);
#35049=AXIS2_PLACEMENT_3D('',#53402,#40700,#40701);
#35050=AXIS2_PLACEMENT_3D('',#53404,#40702,#40703);
#35051=AXIS2_PLACEMENT_3D('',#53407,#40705,#40706);
#35052=AXIS2_PLACEMENT_3D('',#53408,#40707,#40708);
#35053=AXIS2_PLACEMENT_3D('',#53426,#40717,#40718);
#35054=AXIS2_PLACEMENT_3D('',#53434,#40723,#40724);
#35055=AXIS2_PLACEMENT_3D('',#53436,#40725,#40726);
#35056=AXIS2_PLACEMENT_3D('',#53438,#40727,#40728);
#35057=AXIS2_PLACEMENT_3D('',#53440,#40729,#40730);
#35058=AXIS2_PLACEMENT_3D('',#53443,#40732,#40733);
#35059=AXIS2_PLACEMENT_3D('',#53471,#40734,#40735);
#35060=AXIS2_PLACEMENT_3D('',#53499,#40736,#40737);
#35061=AXIS2_PLACEMENT_3D('',#53500,#40738,#40739);
#35062=AXIS2_PLACEMENT_3D('',#53506,#40743,#40744);
#35063=AXIS2_PLACEMENT_3D('',#53509,#40746,#40747);
#35064=AXIS2_PLACEMENT_3D('',#53511,#40749,#40750);
#35065=AXIS2_PLACEMENT_3D('',#53519,#40755,#40756);
#35066=AXIS2_PLACEMENT_3D('',#53521,#40757,#40758);
#35067=AXIS2_PLACEMENT_3D('',#53523,#40759,#40760);
#35068=AXIS2_PLACEMENT_3D('',#53525,#40762,#40763);
#35069=AXIS2_PLACEMENT_3D('',#53527,#40764,#40765);
#35070=AXIS2_PLACEMENT_3D('',#53529,#40766,#40767);
#35071=AXIS2_PLACEMENT_3D('',#53530,#40768,#40769);
#35072=AXIS2_PLACEMENT_3D('',#53531,#40770,#40771);
#35073=AXIS2_PLACEMENT_3D('',#53533,#40772,#40773);
#35074=AXIS2_PLACEMENT_3D('',#53534,#40774,#40775);
#35075=AXIS2_PLACEMENT_3D('',#53535,#40776,#40777);
#35076=AXIS2_PLACEMENT_3D('',#53536,#40778,#40779);
#35077=AXIS2_PLACEMENT_3D('',#53539,#40780,#40781);
#35078=AXIS2_PLACEMENT_3D('',#53541,#40782,#40783);
#35079=AXIS2_PLACEMENT_3D('',#53542,#40784,#40785);
#35080=AXIS2_PLACEMENT_3D('',#53543,#40786,#40787);
#35081=AXIS2_PLACEMENT_3D('',#53546,#40788,#40789);
#35082=AXIS2_PLACEMENT_3D('',#53547,#40790,#40791);
#35083=AXIS2_PLACEMENT_3D('',#53548,#40792,#40793);
#35084=AXIS2_PLACEMENT_3D('',#53549,#40794,#40795);
#35085=AXIS2_PLACEMENT_3D('',#53552,#40796,#40797);
#35086=AXIS2_PLACEMENT_3D('',#53554,#40798,#40799);
#35087=AXIS2_PLACEMENT_3D('',#53555,#40800,#40801);
#35088=AXIS2_PLACEMENT_3D('',#53556,#40802,#40803);
#35089=AXIS2_PLACEMENT_3D('',#53559,#40804,#40805);
#35090=AXIS2_PLACEMENT_3D('',#53560,#40806,#40807);
#35091=AXIS2_PLACEMENT_3D('',#53561,#40808,#40809);
#35092=AXIS2_PLACEMENT_3D('',#53562,#40810,#40811);
#35093=AXIS2_PLACEMENT_3D('',#53565,#40812,#40813);
#35094=AXIS2_PLACEMENT_3D('',#53567,#40814,#40815);
#35095=AXIS2_PLACEMENT_3D('',#53569,#40816,#40817);
#35096=AXIS2_PLACEMENT_3D('',#53570,#40818,#40819);
#35097=AXIS2_PLACEMENT_3D('',#53571,#40820,#40821);
#35098=AXIS2_PLACEMENT_3D('',#53574,#40822,#40823);
#35099=AXIS2_PLACEMENT_3D('',#53575,#40824,#40825);
#35100=AXIS2_PLACEMENT_3D('',#53576,#40826,#40827);
#35101=AXIS2_PLACEMENT_3D('',#53577,#40828,#40829);
#35102=AXIS2_PLACEMENT_3D('',#53580,#40830,#40831);
#35103=AXIS2_PLACEMENT_3D('',#53582,#40832,#40833);
#35104=AXIS2_PLACEMENT_3D('',#53583,#40834,#40835);
#35105=AXIS2_PLACEMENT_3D('',#53584,#40836,#40837);
#35106=AXIS2_PLACEMENT_3D('',#53587,#40838,#40839);
#35107=AXIS2_PLACEMENT_3D('',#53589,#40840,#40841);
#35108=AXIS2_PLACEMENT_3D('',#53590,#40842,#40843);
#35109=AXIS2_PLACEMENT_3D('',#53591,#40844,#40845);
#35110=AXIS2_PLACEMENT_3D('',#53594,#40848,#40849);
#35111=AXIS2_PLACEMENT_3D('',#53597,#40850,#40851);
#35112=AXIS2_PLACEMENT_3D('',#53600,#40854,#40855);
#35113=AXIS2_PLACEMENT_3D('',#53602,#40856,#40857);
#35114=AXIS2_PLACEMENT_3D('',#53604,#40858,#40859);
#35115=AXIS2_PLACEMENT_3D('',#53605,#40860,#40861);
#35116=AXIS2_PLACEMENT_3D('',#53606,#40862,#40863);
#35117=AXIS2_PLACEMENT_3D('',#53608,#40865,#40866);
#35118=AXIS2_PLACEMENT_3D('',#53611,#40869,#40870);
#35119=AXIS2_PLACEMENT_3D('',#53614,#40871,#40872);
#35120=AXIS2_PLACEMENT_3D('',#53615,#40873,#40874);
#35121=AXIS2_PLACEMENT_3D('',#53616,#40875,#40876);
#35122=AXIS2_PLACEMENT_3D('',#53617,#40877,#40878);
#35123=AXIS2_PLACEMENT_3D('',#53619,#40879,#40880);
#35124=AXIS2_PLACEMENT_3D('',#53621,#40882,#40883);
#35125=AXIS2_PLACEMENT_3D('',#53623,#40885,#40886);
#35126=AXIS2_PLACEMENT_3D('',#53626,#40889,#40890);
#35127=AXIS2_PLACEMENT_3D('',#53629,#40893,#40894);
#35128=AXIS2_PLACEMENT_3D('',#53631,#40896,#40897);
#35129=AXIS2_PLACEMENT_3D('',#53634,#40900,#40901);
#35130=AXIS2_PLACEMENT_3D('',#53637,#40904,#40905);
#35131=AXIS2_PLACEMENT_3D('',#53639,#40907,#40908);
#35132=AXIS2_PLACEMENT_3D('',#53642,#40911,#40912);
#35133=AXIS2_PLACEMENT_3D('',#53645,#40915,#40916);
#35134=AXIS2_PLACEMENT_3D('',#53647,#40918,#40919);
#35135=AXIS2_PLACEMENT_3D('',#53650,#40922,#40923);
#35136=AXIS2_PLACEMENT_3D('',#53653,#40926,#40927);
#35137=AXIS2_PLACEMENT_3D('',#53654,#40928,#40929);
#35138=AXIS2_PLACEMENT_3D('',#53656,#40931,#40932);
#35139=AXIS2_PLACEMENT_3D('',#53658,#40933,#40934);
#35140=AXIS2_PLACEMENT_3D('',#53660,#40936,#40937);
#35141=AXIS2_PLACEMENT_3D('',#53667,#40942,#40943);
#35142=AXIS2_PLACEMENT_3D('',#53673,#40947,#40948);
#35143=AXIS2_PLACEMENT_3D('',#53680,#40953,#40954);
#35144=AXIS2_PLACEMENT_3D('',#53682,#40955,#40956);
#35145=AXIS2_PLACEMENT_3D('',#53684,#40957,#40958);
#35146=AXIS2_PLACEMENT_3D('',#53694,#40963,#40964);
#35147=AXIS2_PLACEMENT_3D('',#53696,#40965,#40966);
#35148=AXIS2_PLACEMENT_3D('',#53697,#40967,#40968);
#35149=AXIS2_PLACEMENT_3D('',#53698,#40969,#40970);
#35150=AXIS2_PLACEMENT_3D('',#53699,#40971,#40972);
#35151=AXIS2_PLACEMENT_3D('',#53700,#40973,#40974);
#35152=AXIS2_PLACEMENT_3D('',#53701,#40975,#40976);
#35153=AXIS2_PLACEMENT_3D('',#53703,#40977,#40978);
#35154=AXIS2_PLACEMENT_3D('',#53705,#40980,#40981);
#35155=AXIS2_PLACEMENT_3D('',#53709,#40983,#40984);
#35156=AXIS2_PLACEMENT_3D('',#53710,#40985,#40986);
#35157=AXIS2_PLACEMENT_3D('',#53711,#40987,#40988);
#35158=AXIS2_PLACEMENT_3D('',#53713,#40989,#40990);
#35159=AXIS2_PLACEMENT_3D('',#53715,#40992,#40993);
#35160=AXIS2_PLACEMENT_3D('',#53719,#40995,#40996);
#35161=AXIS2_PLACEMENT_3D('',#53720,#40997,#40998);
#35162=AXIS2_PLACEMENT_3D('',#53721,#40999,#41000);
#35163=AXIS2_PLACEMENT_3D('',#53723,#41001,#41002);
#35164=AXIS2_PLACEMENT_3D('',#53725,#41004,#41005);
#35165=AXIS2_PLACEMENT_3D('',#53729,#41007,#41008);
#35166=AXIS2_PLACEMENT_3D('',#53730,#41009,#41010);
#35167=AXIS2_PLACEMENT_3D('',#53731,#41011,#41012);
#35168=AXIS2_PLACEMENT_3D('',#53733,#41013,#41014);
#35169=AXIS2_PLACEMENT_3D('',#53735,#41016,#41017);
#35170=AXIS2_PLACEMENT_3D('',#53739,#41019,#41020);
#35171=AXIS2_PLACEMENT_3D('',#53740,#41021,#41022);
#35172=AXIS2_PLACEMENT_3D('',#53741,#41023,#41024);
#35173=AXIS2_PLACEMENT_3D('',#53743,#41026,#41027);
#35174=AXIS2_PLACEMENT_3D('',#53745,#41029,#41030);
#35175=AXIS2_PLACEMENT_3D('',#53747,#41032,#41033);
#35176=AXIS2_PLACEMENT_3D('',#53749,#41035,#41036);
#35177=AXIS2_PLACEMENT_3D('',#53751,#41038,#41039);
#35178=AXIS2_PLACEMENT_3D('',#53752,#41040,#41041);
#35179=AXIS2_PLACEMENT_3D('',#53758,#41045,#41046);
#35180=AXIS2_PLACEMENT_3D('',#53760,#41048,#41049);
#35181=AXIS2_PLACEMENT_3D('',#53762,#41051,#41052);
#35182=AXIS2_PLACEMENT_3D('',#53763,#41053,#41054);
#35183=AXIS2_PLACEMENT_3D('',#53767,#41057,#41058);
#35184=AXIS2_PLACEMENT_3D('',#53769,#41060,#41061);
#35185=AXIS2_PLACEMENT_3D('',#53770,#41062,#41063);
#35186=AXIS2_PLACEMENT_3D('',#53772,#41065,#41066);
#35187=AXIS2_PLACEMENT_3D('',#53773,#41067,#41068);
#35188=AXIS2_PLACEMENT_3D('',#53776,#41071,#41072);
#35189=AXIS2_PLACEMENT_3D('',#53778,#41074,#41075);
#35190=AXIS2_PLACEMENT_3D('',#53780,#41077,#41078);
#40665=DIRECTION('axis',(0.,0.,1.));
#40666=DIRECTION('refdir',(1.,0.,0.));
#40667=DIRECTION('center_axis',(1.,-5.00596043936353E-16,-3.34404360992166E-15));
#40668=DIRECTION('ref_axis',(-2.71857077046111E-15,-0.707106781186757,-0.707106781186338));
#40669=DIRECTION('center_axis',(-1.,5.00596043936353E-16,3.34404360992166E-15));
#40670=DIRECTION('ref_axis',(-2.71857077046111E-15,-0.707106781186757,-0.707106781186338));
#40671=DIRECTION('',(1.,-5.00596043936353E-16,-3.34404360992166E-15));
#40672=DIRECTION('center_axis',(1.,-5.00596043936353E-16,-3.34404360992166E-15));
#40673=DIRECTION('ref_axis',(-2.71857077046111E-15,-0.707106781186757,-0.707106781186338));
#40674=DIRECTION('',(-1.,5.00596043936353E-16,3.34404360992166E-15));
#40675=DIRECTION('center_axis',(-3.34404360992166E-15,5.94374044734026E-16,
-1.));
#40676=DIRECTION('ref_axis',(5.00596043936355E-16,1.,5.94374044734051E-16));
#40677=DIRECTION('',(5.00596043936355E-16,1.,5.94374044734026E-16));
#40678=DIRECTION('',(-1.,5.00596043936353E-16,3.34404360992166E-15));
#40679=DIRECTION('',(-5.00596043936355E-16,-1.,-5.94374044734026E-16));
#40680=DIRECTION('',(1.,-5.00596043936353E-16,-3.34404360992166E-15));
#40681=DIRECTION('',(5.00596043936355E-16,1.,5.94374044734026E-16));
#40682=DIRECTION('',(-1.,5.00596043936353E-16,3.34404360992166E-15));
#40683=DIRECTION('',(-5.00596043936355E-16,-1.,-5.94374044734026E-16));
#40684=DIRECTION('',(1.,-5.00596043936353E-16,-3.34404360992166E-15));
#40685=DIRECTION('',(5.00596043936355E-16,1.,5.94374044734026E-16));
#40686=DIRECTION('',(-1.,5.00596043936353E-16,3.34404360992166E-15));
#40687=DIRECTION('',(-5.00596043936355E-16,-1.,-5.94374044734026E-16));
#40688=DIRECTION('center_axis',(-3.34404360992166E-15,5.94374044734026E-16,
-1.));
#40689=DIRECTION('ref_axis',(-5.00596043936355E-16,-1.,-5.94374044734082E-16));
#40690=DIRECTION('center_axis',(-3.34404360992166E-15,5.94374044734026E-16,
-1.));
#40691=DIRECTION('ref_axis',(-5.00596043936355E-16,-1.,-5.94374044734082E-16));
#40692=DIRECTION('',(-1.,5.00596043936353E-16,3.34404360992166E-15));
#40693=DIRECTION('',(-5.00596043936355E-16,-1.,-5.94374044734026E-16));
#40694=DIRECTION('',(1.,-5.00596043936353E-16,-3.34404360992166E-15));
#40695=DIRECTION('',(5.00596043936355E-16,1.,5.94374044734026E-16));
#40696=DIRECTION('center_axis',(-3.34404360992166E-15,5.94374044734026E-16,
-1.));
#40697=DIRECTION('ref_axis',(-5.00596043936355E-16,-1.,-5.94374044734082E-16));
#40698=DIRECTION('center_axis',(-3.34404360992166E-15,5.94374044734026E-16,
-1.));
#40699=DIRECTION('ref_axis',(-5.00596043936355E-16,-1.,-5.94374044734082E-16));
#40700=DIRECTION('center_axis',(-5.00596043936355E-16,-1.,-5.94374044734026E-16));
#40701=DIRECTION('ref_axis',(0.707106781186527,6.63110602902038E-17,-0.707106781186568));
#40702=DIRECTION('center_axis',(5.00596043936355E-16,1.,6.19091582356982E-16));
#40703=DIRECTION('ref_axis',(0.707106781186527,8.37889987576735E-17,-0.707106781186568));
#40704=DIRECTION('',(-5.00596043936355E-16,-1.,-5.94374044734026E-16));
#40705=DIRECTION('center_axis',(-5.00596043936355E-16,-1.,-5.94374044734026E-16));
#40706=DIRECTION('ref_axis',(0.707106781186527,6.63110602902038E-17,-0.707106781186568));
#40707=DIRECTION('center_axis',(1.,-5.00596043936353E-16,-3.34404360992166E-15));
#40708=DIRECTION('ref_axis',(-5.00596043934382E-16,-1.,5.89417440552492E-13));
#40709=DIRECTION('',(-3.34404360992166E-15,5.94374044734026E-16,-1.));
#40710=DIRECTION('',(-3.34404360992166E-15,6.19091582356982E-16,-1.));
#40711=DIRECTION('',(5.00596043931499E-16,1.,-1.45135967092772E-12));
#40712=DIRECTION('',(-3.34404360992166E-15,6.19091582356982E-16,-1.));
#40713=DIRECTION('',(1.01071973798223E-15,-0.899510317025162,0.436899518843055));
#40714=DIRECTION('',(-5.005960439315E-16,-1.,1.45135967092772E-12));
#40715=DIRECTION('',(-3.34404360992195E-15,-5.89417440552492E-13,-1.));
#40716=DIRECTION('',(5.00596043930822E-16,1.,-1.65391127897018E-12));
#40717=DIRECTION('center_axis',(1.,-5.00596043936353E-16,-3.34404360992166E-15));
#40718=DIRECTION('ref_axis',(-3.37116090328259E-15,-0.224153611366395,-0.974553825353635));
#40719=DIRECTION('',(-1.01071973799428E-15,0.899510317023531,-0.436899518846413));
#40720=DIRECTION('',(5.00596043934382E-16,1.,-5.89417440552492E-13));
#40721=DIRECTION('',(3.34404360992195E-15,5.89417440552492E-13,1.));
#40722=DIRECTION('',(5.00596043931499E-16,1.,-1.45135967092772E-12));
#40723=DIRECTION('center_axis',(1.,-5.00596043936353E-16,-3.34404360992166E-15));
#40724=DIRECTION('ref_axis',(3.37116090328329E-15,0.224153611363817,0.974553825354228));
#40725=DIRECTION('center_axis',(-1.,5.00596043936353E-16,3.34404360992166E-15));
#40726=DIRECTION('ref_axis',(3.37116090328329E-15,0.224153611363817,0.974553825354228));
#40727=DIRECTION('center_axis',(1.,-5.00596043936353E-16,-3.34404360992166E-15));
#40728=DIRECTION('ref_axis',(3.37116090328329E-15,0.224153611363817,0.974553825354228));
#40729=DIRECTION('center_axis',(-1.,-1.77856601184676E-14,1.22258278069232E-14));
#40730=DIRECTION('ref_axis',(1.22258278069229E-14,2.09832519444149E-14,
1.));
#40731=DIRECTION('',(1.,-5.00596043936353E-16,-3.34404360992166E-15));
#40732=DIRECTION('center_axis',(1.,-5.00596043936353E-16,-3.34404360992166E-15));
#40733=DIRECTION('ref_axis',(3.22671189843719E-15,0.436899518843004,0.899510317025186));
#40734=DIRECTION('center_axis',(1.50162002879617E-14,-0.436899518843088,
-0.899510317025146));
#40735=DIRECTION('ref_axis',(5.31748758588635E-11,0.899510317025146,-0.436899518843088));
#40736=DIRECTION('center_axis',(1.70009668144121E-14,-0.436899518843016,
-0.899510317025181));
#40737=DIRECTION('ref_axis',(-3.85139127936184E-11,0.89951031702518,-0.436899518843016));
#40738=DIRECTION('center_axis',(-1.,5.00596043936353E-16,3.34404360992166E-15));
#40739=DIRECTION('ref_axis',(5.00596043936355E-16,1.,6.88301496270999E-16));
#40740=DIRECTION('',(-3.34404360992166E-15,6.19091582356982E-16,-1.));
#40741=DIRECTION('',(-5.00596043931499E-16,-1.,1.45135967092772E-12));
#40742=DIRECTION('',(-3.34404360992166E-15,6.19091582356982E-16,-1.));
#40743=DIRECTION('center_axis',(5.00596043936355E-16,1.,6.19091582356982E-16));
#40744=DIRECTION('ref_axis',(1.,-5.00596043936353E-16,-3.34404360992166E-15));
#40745=DIRECTION('',(1.,-5.00596043936353E-16,-3.34404360992166E-15));
#40746=DIRECTION('center_axis',(-5.00596043936355E-16,-1.,-6.19091582356982E-16));
#40747=DIRECTION('ref_axis',(-4.15545247511164E-15,6.19091582356955E-16,
-1.));
#40748=DIRECTION('',(-1.,5.00596043936353E-16,3.34404360992166E-15));
#40749=DIRECTION('center_axis',(-3.22671189843713E-15,-0.436899518843055,
-0.899510317025162));
#40750=DIRECTION('ref_axis',(-1.01071973798224E-15,0.899510317025162,-0.436899518843055));
#40751=DIRECTION('',(1.,-5.00596043936353E-16,-3.34404360992166E-15));
#40752=DIRECTION('',(1.01071973798224E-15,-0.899510317025162,0.436899518843055));
#40753=DIRECTION('',(-1.,5.00596043936353E-16,3.34404360992166E-15));
#40754=DIRECTION('',(-1.01071973798223E-15,0.899510317025162,-0.436899518843055));
#40755=DIRECTION('center_axis',(-5.00596043936355E-16,-1.,-5.94374044734026E-16));
#40756=DIRECTION('ref_axis',(-0.707106781186548,7.74260774895239E-16,-0.707106781186547));
#40757=DIRECTION('center_axis',(5.00596043936355E-16,1.,6.19091582357991E-16));
#40758=DIRECTION('ref_axis',(-0.707106781186548,7.91738713363403E-16,-0.707106781186547));
#40759=DIRECTION('center_axis',(-5.00596043936355E-16,-1.,-5.94374044734026E-16));
#40760=DIRECTION('ref_axis',(-0.707106781186548,7.74260774895239E-16,-0.707106781186547));
#40761=DIRECTION('',(5.00596043936355E-16,1.,5.94374044734026E-16));
#40762=DIRECTION('center_axis',(0.0929057196031524,-0.979910694923634,0.176475372897471));
#40763=DIRECTION('ref_axis',(-0.456482036021868,-0.199436781899079,-0.867092336960182));
#40764=DIRECTION('center_axis',(-1.0107197379821E-15,0.89951031702518,-0.436899518843017));
#40765=DIRECTION('ref_axis',(-1.,5.00596043936353E-16,3.34404360992166E-15));
#40766=DIRECTION('center_axis',(-5.00596043931531E-16,-1.,1.44206872346462E-12));
#40767=DIRECTION('ref_axis',(-3.34404360992238E-15,-1.44206872346462E-12,
-1.));
#40768=DIRECTION('center_axis',(-1.,5.00596043936353E-16,3.34404360992166E-15));
#40769=DIRECTION('ref_axis',(-3.22671189843719E-15,-0.436899518843004,-0.899510317025186));
#40770=DIRECTION('center_axis',(-0.0929057196030986,-0.979910694923638,
0.176475372897477));
#40771=DIRECTION('ref_axis',(0.456482036021868,-0.199436781899079,-0.867092336960182));
#40772=DIRECTION('center_axis',(1.,-5.00596043936353E-16,-3.34404360992166E-15));
#40773=DIRECTION('ref_axis',(-3.34404360992238E-15,-1.44206872346462E-12,
-1.));
#40774=DIRECTION('center_axis',(-5.00596043931531E-16,-1.,1.44206872346462E-12));
#40775=DIRECTION('ref_axis',(1.,-5.00596043936353E-16,-3.34404360992166E-15));
#40776=DIRECTION('center_axis',(-1.01071973798204E-15,0.899510317025188,
-0.436899518843));
#40777=DIRECTION('ref_axis',(-3.22671189843719E-15,-0.436899518843,-0.899510317025188));
#40778=DIRECTION('center_axis',(-0.408248290464166,0.408248290464166,0.816496580927423));
#40779=DIRECTION('ref_axis',(-0.577350269189777,0.577350269188982,-0.577350269190118));
#40780=DIRECTION('center_axis',(5.00596043931531E-16,1.,-1.44206872346462E-12));
#40781=DIRECTION('ref_axis',(-1.,5.00596043936353E-16,3.34404360992166E-15));
#40782=DIRECTION('center_axis',(-3.34404360992196E-15,-5.89417440552492E-13,
-1.));
#40783=DIRECTION('ref_axis',(5.00596043934382E-16,1.,-5.89417440552492E-13));
#40784=DIRECTION('center_axis',(-1.,5.00596043936353E-16,3.34404360992166E-15));
#40785=DIRECTION('ref_axis',(-3.34404360992238E-15,-1.44206872346462E-12,
-1.));
#40786=DIRECTION('center_axis',(0.408248290463598,-0.816496580928219,-0.408248290463143));
#40787=DIRECTION('ref_axis',(0.577350269189777,0.577350269188982,-0.577350269190118));
#40788=DIRECTION('center_axis',(1.,-5.00596043936353E-16,-3.34404360992166E-15));
#40789=DIRECTION('ref_axis',(5.00596043934382E-16,1.,-5.89417440552492E-13));
#40790=DIRECTION('center_axis',(-3.34404360992196E-15,-5.89417440552492E-13,
-1.));
#40791=DIRECTION('ref_axis',(1.,-5.00596043936353E-16,-3.34404360992166E-15));
#40792=DIRECTION('center_axis',(5.00596043931531E-16,1.,-1.44206872346462E-12));
#40793=DIRECTION('ref_axis',(-3.34404360992238E-15,-1.44206872346462E-12,
-1.));
#40794=DIRECTION('center_axis',(0.816496580927953,0.408248290464147,0.408248290463124));
#40795=DIRECTION('ref_axis',(-0.577350269189285,0.577350269190592,0.577350269189001));
#40796=DIRECTION('center_axis',(3.34404360992196E-15,5.89417440552492E-13,
1.));
#40797=DIRECTION('ref_axis',(-1.,5.00596043936353E-16,3.34404360992166E-15));
#40798=DIRECTION('center_axis',(2.84717690347971E-13,1.,-1.72628581776865E-12));
#40799=DIRECTION('ref_axis',(3.34404360992252E-15,1.72628581776865E-12,
1.));
#40800=DIRECTION('center_axis',(-1.,5.00596043936353E-16,3.34404360992166E-15));
#40801=DIRECTION('ref_axis',(5.00596043934382E-16,1.,-5.89417440552492E-13));
#40802=DIRECTION('center_axis',(0.81649658092784,-0.408248290464147,-0.408248290463351));
#40803=DIRECTION('ref_axis',(0.577350269189436,0.577350269190346,0.577350269189095));
#40804=DIRECTION('center_axis',(1.,-5.00596043936353E-16,-3.34404360992166E-15));
#40805=DIRECTION('ref_axis',(3.34404360992252E-15,1.72628581776865E-12,
1.));
#40806=DIRECTION('center_axis',(5.00596043931531E-16,1.,-1.44206872346462E-12));
#40807=DIRECTION('ref_axis',(1.,-5.00596043936353E-16,-3.34404360992166E-15));
#40808=DIRECTION('center_axis',(3.34404360992196E-15,5.89417440552492E-13,
1.));
#40809=DIRECTION('ref_axis',(5.00596043934382E-16,1.,-5.89417440552492E-13));
#40810=DIRECTION('center_axis',(-1.,5.00596043936353E-16,3.34404360992166E-15));
#40811=DIRECTION('ref_axis',(0.,1.,-5.68434188608075E-13));
#40812=DIRECTION('center_axis',(-1.,5.00596043936353E-16,3.34404360992166E-15));
#40813=DIRECTION('ref_axis',(-3.3711609032826E-15,-0.224153611366396,-0.974553825353635));
#40814=DIRECTION('center_axis',(1.01071973799424E-15,-0.899510317023536,
0.436899518846402));
#40815=DIRECTION('ref_axis',(3.22671189843337E-15,0.436899518846402,0.899510317023536));
#40816=DIRECTION('center_axis',(1.,-5.00596043936353E-16,-3.34404360992166E-15));
#40817=DIRECTION('ref_axis',(-3.34404360992245E-15,-1.58417727061664E-12,
-1.));
#40818=DIRECTION('center_axis',(5.00596043931055E-16,1.,-1.58417727061664E-12));
#40819=DIRECTION('ref_axis',(-1.,5.00596043936353E-16,3.34404360992166E-15));
#40820=DIRECTION('center_axis',(-1.,5.00596043936353E-16,3.34404360992166E-15));
#40821=DIRECTION('ref_axis',(0.,1.,-5.6843418860808E-13));
#40822=DIRECTION('center_axis',(-1.,5.00596043936353E-16,3.34404360992166E-15));
#40823=DIRECTION('ref_axis',(-3.22671189843335E-15,-0.436899518846416,-0.899510317023529));
#40824=DIRECTION('center_axis',(1.01071973799427E-15,-0.899510317023533,
0.436899518846409));
#40825=DIRECTION('ref_axis',(1.,-5.00596043936353E-16,-3.34404360992166E-15));
#40826=DIRECTION('center_axis',(5.00596043931055E-16,1.,-1.58417727061664E-12));
#40827=DIRECTION('ref_axis',(3.34404360992245E-15,1.58417727061664E-12,
1.));
#40828=DIRECTION('center_axis',(-0.0929057196037775,-0.97991069492339,0.176475372898494));
#40829=DIRECTION('ref_axis',(-0.456482036022069,0.199436781900318,0.867092336959791));
#40830=DIRECTION('center_axis',(1.01071973799424E-15,-0.899510317023537,
0.4368995188464));
#40831=DIRECTION('ref_axis',(-1.,5.00596043936353E-16,3.34404360992166E-15));
#40832=DIRECTION('center_axis',(5.00596043934382E-16,1.,-5.89417440552492E-13));
#40833=DIRECTION('ref_axis',(3.34404360992196E-15,5.89417440552492E-13,
1.));
#40834=DIRECTION('center_axis',(-1.,5.00596043936353E-16,3.34404360992166E-15));
#40835=DIRECTION('ref_axis',(3.22671189843336E-15,0.436899518846405,0.899510317023535));
#40836=DIRECTION('center_axis',(0.816496580927783,-0.408248290463579,0.408248290464034));
#40837=DIRECTION('ref_axis',(-0.577350269189588,-0.577350269189304,0.577350269189986));
#40838=DIRECTION('center_axis',(-1.,5.00596043936353E-16,3.34404360992166E-15));
#40839=DIRECTION('ref_axis',(3.34404360992196E-15,5.89417440552492E-13,
1.));
#40840=DIRECTION('center_axis',(-5.00596043934382E-16,-1.,5.89417440552492E-13));
#40841=DIRECTION('ref_axis',(-1.,5.00596043936353E-16,3.34404360992166E-15));
#40842=DIRECTION('center_axis',(-1.09684848857867E-15,5.89417440552492E-13,
1.));
#40843=DIRECTION('ref_axis',(-5.00596043934382E-16,-1.,5.89417440552492E-13));
#40844=DIRECTION('center_axis',(5.00596043934382E-16,1.,-5.89417440552492E-13));
#40845=DIRECTION('ref_axis',(-0.707106781186544,4.17135044021589E-13,0.707106781186551));
#40846=DIRECTION('',(-5.00596043934382E-16,-1.,5.89417440552492E-13));
#40847=DIRECTION('',(5.00596043934382E-16,1.,-5.89417440552492E-13));
#40848=DIRECTION('center_axis',(3.34404360992196E-15,5.89417440552492E-13,
1.));
#40849=DIRECTION('ref_axis',(-0.707106781186543,-0.707106781186552,4.19145665077448E-13));
#40850=DIRECTION('center_axis',(3.34404360992239E-15,1.45135967092772E-12,
1.));
#40851=DIRECTION('ref_axis',(-0.707106781186543,-0.707106781186552,1.02863086116683E-12));
#40852=DIRECTION('',(3.34404360992196E-15,5.89417440552492E-13,1.));
#40853=DIRECTION('',(-3.34404360992196E-15,-5.89417440552492E-13,-1.));
#40854=DIRECTION('center_axis',(0.0929057196037781,-0.97991069492339,0.176475372898495));
#40855=DIRECTION('ref_axis',(0.456482036022066,0.199436781900346,0.867092336959786));
#40856=DIRECTION('center_axis',(5.00596043934382E-16,1.,-5.89417440552492E-13));
#40857=DIRECTION('ref_axis',(1.,-5.00596043936353E-16,-3.34404360992166E-15));
#40858=DIRECTION('center_axis',(4.89116698015727E-15,-0.899510317023533,
0.436899518846409));
#40859=DIRECTION('ref_axis',(3.22671189843336E-15,0.436899518846409,0.899510317023533));
#40860=DIRECTION('center_axis',(1.,-5.00596043936353E-16,-3.34404360992166E-15));
#40861=DIRECTION('ref_axis',(3.34404360992196E-15,5.89417440552492E-13,
1.));
#40862=DIRECTION('center_axis',(-1.01071973799428E-15,0.899510317023531,
-0.436899518846413));
#40863=DIRECTION('ref_axis',(0.707106781186553,0.308934612473437,0.636049844914594));
#40864=DIRECTION('',(1.01071973799428E-15,-0.899510317023531,0.436899518846413));
#40865=DIRECTION('center_axis',(1.,-5.00596043936353E-16,-3.34404360992166E-15));
#40866=DIRECTION('ref_axis',(3.37116090328272E-15,0.22415361136594,0.974553825353739));
#40867=DIRECTION('',(-1.,5.00596043936353E-16,3.34404360992166E-15));
#40868=DIRECTION('',(1.,-5.00596043936353E-16,-3.34404360992166E-15));
#40869=DIRECTION('center_axis',(-0.408248290463825,-0.816496580927991,-0.40824829046337));
#40870=DIRECTION('ref_axis',(0.577350269189588,-0.577350269189247,0.577350269190043));
#40871=DIRECTION('center_axis',(1.,-5.00596043936353E-16,-3.34404360992166E-15));
#40872=DIRECTION('ref_axis',(-5.00596043934382E-16,-1.,5.89417440552492E-13));
#40873=DIRECTION('center_axis',(3.34404360992196E-15,5.98299224749493E-13,
1.));
#40874=DIRECTION('ref_axis',(1.,-5.00596043936353E-16,-3.34404360992166E-15));
#40875=DIRECTION('center_axis',(-5.00596043934382E-16,-1.,5.89417440552492E-13));
#40876=DIRECTION('ref_axis',(3.34404360992196E-15,5.89417440552492E-13,
1.));
#40877=DIRECTION('center_axis',(-3.34404360992195E-15,-5.89417440552492E-13,
-1.));
#40878=DIRECTION('ref_axis',(0.707106781186522,-0.707106781186573,4.14416473251142E-13));
#40879=DIRECTION('center_axis',(3.34404360992239E-15,1.45135967092772E-12,
1.));
#40880=DIRECTION('ref_axis',(0.707106781186522,-0.707106781186573,1.02390166934054E-12));
#40881=DIRECTION('',(-3.34404360992195E-15,-5.89417440552492E-13,-1.));
#40882=DIRECTION('center_axis',(5.00596043934382E-16,1.,-5.89417440552492E-13));
#40883=DIRECTION('ref_axis',(0.707106781186528,4.16427094306996E-13,0.707106781186567));
#40884=DIRECTION('',(-5.00596043934382E-16,-1.,5.89417440552492E-13));
#40885=DIRECTION('center_axis',(1.,-5.00596043936353E-16,-3.34404360992166E-15));
#40886=DIRECTION('ref_axis',(2.01062105585817E-15,-0.707106781186137,0.707106781186958));
#40887=DIRECTION('',(-1.,5.00596043936353E-16,3.34404360992166E-15));
#40888=DIRECTION('',(1.,-5.00596043936353E-16,-3.34404360992166E-15));
#40889=DIRECTION('center_axis',(-1.01071973799428E-15,0.899510317023531,
-0.436899518846413));
#40890=DIRECTION('ref_axis',(-0.707106781186563,0.308934612473431,0.636049844914586));
#40891=DIRECTION('',(1.01071973799428E-15,-0.899510317023531,0.436899518846413));
#40892=DIRECTION('',(-1.01071973799428E-15,0.899510317023531,-0.436899518846413));
#40893=DIRECTION('center_axis',(5.00596043930822E-16,1.,-1.65391127897018E-12));
#40894=DIRECTION('ref_axis',(0.707106781186531,1.16913790598346E-12,0.707106781186564));
#40895=DIRECTION('',(-5.00596043930822E-16,-1.,1.65391127897018E-12));
#40896=DIRECTION('center_axis',(1.,-5.00596043936353E-16,-3.34404360992166E-15));
#40897=DIRECTION('ref_axis',(-3.37116090328261E-15,-0.224153611366358,-0.974553825353643));
#40898=DIRECTION('',(-1.,5.00596043936353E-16,3.34404360992166E-15));
#40899=DIRECTION('',(1.,-5.00596043936353E-16,-3.34404360992166E-15));
#40900=DIRECTION('center_axis',(5.00596043930822E-16,1.,-1.65391127897018E-12));
#40901=DIRECTION('ref_axis',(-0.707106781186547,1.16984585569803E-12,0.707106781186548));
#40902=DIRECTION('',(-5.00596043930822E-16,-1.,1.65391127897018E-12));
#40903=DIRECTION('',(5.00596043930822E-16,1.,-1.65391127897018E-12));
#40904=DIRECTION('center_axis',(-3.34404360992195E-15,-5.89417440552492E-13,
-1.));
#40905=DIRECTION('ref_axis',(0.707106781186648,0.707106781186447,-4.19145665077386E-13));
#40906=DIRECTION('',(3.34404360992195E-15,5.89417440552492E-13,1.));
#40907=DIRECTION('center_axis',(1.,-5.00596043936353E-16,-3.34404360992166E-15));
#40908=DIRECTION('ref_axis',(2.71857077045914E-15,0.707106781187448,0.707106781185647));
#40909=DIRECTION('',(-1.,5.00596043936353E-16,3.34404360992166E-15));
#40910=DIRECTION('',(1.,-5.00596043936353E-16,-3.34404360992166E-15));
#40911=DIRECTION('center_axis',(-3.34404360992196E-15,-5.89417440552492E-13,
-1.));
#40912=DIRECTION('ref_axis',(-0.707106781186668,0.707106781186427,-4.14416473251055E-13));
#40913=DIRECTION('',(3.34404360992196E-15,5.89417440552492E-13,1.));
#40914=DIRECTION('',(-3.34404360992196E-15,-5.89417440552492E-13,-1.));
#40915=DIRECTION('center_axis',(-5.005960439315E-16,-1.,1.45135967092772E-12));
#40916=DIRECTION('ref_axis',(0.707106781186527,-1.026620240111E-12,-0.707106781186568));
#40917=DIRECTION('',(5.005960439315E-16,1.,-1.45135967092772E-12));
#40918=DIRECTION('center_axis',(1.,-5.00596043936353E-16,-3.34404360992166E-15));
#40919=DIRECTION('ref_axis',(-2.01062105585943E-15,0.70710678118581,-0.707106781187285));
#40920=DIRECTION('',(-1.,5.00596043936353E-16,3.34404360992166E-15));
#40921=DIRECTION('',(1.,-5.00596043936353E-16,-3.34404360992166E-15));
#40922=DIRECTION('center_axis',(-5.00596043931499E-16,-1.,1.45135967092772E-12));
#40923=DIRECTION('ref_axis',(-0.707106781186551,-1.02591229039636E-12,-0.707106781186544));
#40924=DIRECTION('',(5.00596043931499E-16,1.,-1.45135967092772E-12));
#40925=DIRECTION('',(-5.00596043931499E-16,-1.,1.45135967092772E-12));
#40926=DIRECTION('center_axis',(1.01071973798223E-15,-0.899510317025162,
0.436899518843055));
#40927=DIRECTION('ref_axis',(0.707106781186558,-0.308934612471059,-0.636049844915743));
#40928=DIRECTION('center_axis',(1.,-5.00596043936353E-16,-3.34404360992166E-15));
#40929=DIRECTION('ref_axis',(-3.3711609032831E-15,-0.224153611364509,-0.974553825354069));
#40930=DIRECTION('',(1.,-5.00596043936353E-16,-3.34404360992166E-15));
#40931=DIRECTION('center_axis',(1.01071973798224E-15,-0.899510317025162,
0.436899518843055));
#40932=DIRECTION('ref_axis',(-0.70710678118655,-0.308934612471064,-0.63604984491575));
#40933=DIRECTION('center_axis',(-5.00596043936355E-16,-1.,-6.19091582357991E-16));
#40934=DIRECTION('ref_axis',(-2.96954721060321E-15,6.19091582357976E-16,
-1.));
#40935=DIRECTION('',(-1.01071973798224E-15,0.899510317025162,-0.436899518843055));
#40936=DIRECTION('center_axis',(-5.00596043934382E-16,-1.,5.89417440552492E-13));
#40937=DIRECTION('ref_axis',(-3.34404360992196E-15,-5.89417440552492E-13,
-1.));
#40938=DIRECTION('',(-3.34404360992166E-15,5.94374044734026E-16,-1.));
#40939=DIRECTION('',(1.,-1.44934907093772E-13,-3.34404360971203E-15));
#40940=DIRECTION('',(1.,-5.00596043936353E-16,-3.34404360992166E-15));
#40941=DIRECTION('',(-3.34404360992166E-15,5.94374044734026E-16,-1.));
#40942=DIRECTION('center_axis',(-3.34404360992239E-15,-1.45135967092772E-12,
-1.));
#40943=DIRECTION('ref_axis',(-1.,5.00596043936353E-16,3.34404360992166E-15));
#40944=DIRECTION('',(-5.00596043931499E-16,-1.,1.45135967092772E-12));
#40945=DIRECTION('',(-1.,5.00596043936353E-16,3.34404360992166E-15));
#40946=DIRECTION('',(5.00596043931499E-16,1.,-1.45135967092772E-12));
#40947=DIRECTION('center_axis',(-1.,5.00596043936353E-16,3.34404360992166E-15));
#40948=DIRECTION('ref_axis',(5.00596043934382E-16,1.,-5.89417440552492E-13));
#40949=DIRECTION('',(-3.34404360992166E-15,5.94374044734026E-16,-1.));
#40950=DIRECTION('',(-3.34404360992166E-15,6.19091582358092E-16,-1.));
#40951=DIRECTION('',(-5.00596043931499E-16,-1.,1.45135967092772E-12));
#40952=DIRECTION('',(-3.34404360992166E-15,6.19091582358092E-16,-1.));
#40953=DIRECTION('center_axis',(3.34404360992196E-15,5.89417440552492E-13,
1.));
#40954=DIRECTION('ref_axis',(-5.00596043934382E-16,-1.,5.89417440552492E-13));
#40955=DIRECTION('center_axis',(3.34404360992196E-15,5.89417440552492E-13,
1.));
#40956=DIRECTION('ref_axis',(5.00596043934382E-16,1.,-5.89417440552492E-13));
#40957=DIRECTION('center_axis',(3.34404360992196E-15,5.89417440552492E-13,
1.));
#40958=DIRECTION('ref_axis',(5.00596043934382E-16,1.,-5.89417440552492E-13));
#40959=DIRECTION('',(1.,-5.00596043936353E-16,-3.34404360992166E-15));
#40960=DIRECTION('',(-5.00596043934382E-16,-1.,5.89417440552492E-13));
#40961=DIRECTION('',(-1.,5.00596043936353E-16,3.34404360992166E-15));
#40962=DIRECTION('',(5.00596043934382E-16,1.,-5.89417440552492E-13));
#40963=DIRECTION('center_axis',(3.34404360992196E-15,5.89417440552492E-13,
1.));
#40964=DIRECTION('ref_axis',(5.00596043934382E-16,1.,-5.89417440552492E-13));
#40965=DIRECTION('center_axis',(3.34404360992196E-15,5.89417440552492E-13,
1.));
#40966=DIRECTION('ref_axis',(5.00596043934382E-16,1.,-5.89417440552492E-13));
#40967=DIRECTION('center_axis',(3.22671189843335E-15,0.436899518846413,
0.899510317023531));
#40968=DIRECTION('ref_axis',(1.01071973799428E-15,-0.899510317023531,0.436899518846413));
#40969=DIRECTION('center_axis',(3.34404360992249E-15,1.65391127897018E-12,
1.));
#40970=DIRECTION('ref_axis',(-5.00596043930822E-16,-1.,1.65391127897018E-12));
#40971=DIRECTION('center_axis',(5.00596043934382E-16,1.,-5.89417440552492E-13));
#40972=DIRECTION('ref_axis',(3.34404360992196E-15,5.89417440552492E-13,
1.));
#40973=DIRECTION('center_axis',(-3.34404360992239E-15,-1.45135967092772E-12,
-1.));
#40974=DIRECTION('ref_axis',(5.005960439315E-16,1.,-1.45135967092772E-12));
#40975=DIRECTION('center_axis',(3.34404360992196E-15,5.89417440552492E-13,
1.));
#40976=DIRECTION('ref_axis',(5.00596043934382E-16,1.,-5.89417440552492E-13));
#40977=DIRECTION('center_axis',(-3.34404360992196E-15,-5.89417440552492E-13,
-1.));
#40978=DIRECTION('ref_axis',(5.00596043934382E-16,1.,-5.89417440552492E-13));
#40979=DIRECTION('',(2.09721666198178E-15,-0.707106781051793,0.707106781321302));
#40980=DIRECTION('center_axis',(-3.34404360992166E-15,5.94374044734026E-16,
-1.));
#40981=DIRECTION('ref_axis',(5.00596043936355E-16,1.,5.94374044734015E-16));
#40982=DIRECTION('',(-3.34404360992166E-15,5.94374044734026E-16,-1.));
#40983=DIRECTION('center_axis',(3.34404360992166E-15,-5.94374044734026E-16,
1.));
#40984=DIRECTION('ref_axis',(-5.00596043936355E-16,-1.,-5.94374044734015E-16));
#40985=DIRECTION('center_axis',(3.34404360992166E-15,-5.94374044734026E-16,
1.));
#40986=DIRECTION('ref_axis',(-5.00596043936355E-16,-1.,-5.94374044734015E-16));
#40987=DIRECTION('center_axis',(3.34404360992196E-15,5.89417440552492E-13,
1.));
#40988=DIRECTION('ref_axis',(5.00596043934382E-16,1.,-5.89417440552492E-13));
#40989=DIRECTION('center_axis',(-3.34404360992196E-15,-5.89417440552492E-13,
-1.));
#40990=DIRECTION('ref_axis',(5.00596043934382E-16,1.,-5.89417440552492E-13));
#40991=DIRECTION('',(2.09721666164013E-15,-0.707106781143578,0.707106781229517));
#40992=DIRECTION('center_axis',(-3.34404360992166E-15,5.94374044734026E-16,
-1.));
#40993=DIRECTION('ref_axis',(5.00596043936355E-16,1.,5.94374044734015E-16));
#40994=DIRECTION('',(-3.34404360992166E-15,5.94374044734026E-16,-1.));
#40995=DIRECTION('center_axis',(3.34404360992166E-15,-5.94374044734026E-16,
1.));
#40996=DIRECTION('ref_axis',(-5.00596043936355E-16,-1.,-5.94374044734015E-16));
#40997=DIRECTION('center_axis',(3.34404360992166E-15,-5.94374044734026E-16,
1.));
#40998=DIRECTION('ref_axis',(-5.00596043936355E-16,-1.,-5.94374044734015E-16));
#40999=DIRECTION('center_axis',(3.34404360992196E-15,5.89417440552492E-13,
1.));
#41000=DIRECTION('ref_axis',(5.00596043934382E-16,1.,-5.89417440552492E-13));
#41001=DIRECTION('center_axis',(-3.34404360992196E-15,-5.89417440552492E-13,
-1.));
#41002=DIRECTION('ref_axis',(5.00596043934382E-16,1.,-5.89417440552492E-13));
#41003=DIRECTION('',(2.09721666164013E-15,-0.707106781143578,0.707106781229517));
#41004=DIRECTION('center_axis',(-3.34404360992166E-15,5.94374044734026E-16,
-1.));
#41005=DIRECTION('ref_axis',(5.00596043936355E-16,1.,5.94374044734015E-16));
#41006=DIRECTION('',(-3.34404360992166E-15,5.94374044734026E-16,-1.));
#41007=DIRECTION('center_axis',(3.34404360992166E-15,-5.94374044734026E-16,
1.));
#41008=DIRECTION('ref_axis',(-5.00596043936355E-16,-1.,-5.94374044734015E-16));
#41009=DIRECTION('center_axis',(3.34404360992166E-15,-5.94374044734026E-16,
1.));
#41010=DIRECTION('ref_axis',(-5.00596043936355E-16,-1.,-5.94374044734015E-16));
#41011=DIRECTION('center_axis',(3.34404360992196E-15,5.89417440552492E-13,
1.));
#41012=DIRECTION('ref_axis',(5.00596043934382E-16,1.,-5.89417440552492E-13));
#41013=DIRECTION('center_axis',(-3.34404360992196E-15,-5.89417440552492E-13,
-1.));
#41014=DIRECTION('ref_axis',(5.00596043934382E-16,1.,-5.89417440552492E-13));
#41015=DIRECTION('',(2.09721666198178E-15,-0.707106781051793,0.707106781321302));
#41016=DIRECTION('center_axis',(-3.34404360992166E-15,5.94374044734026E-16,
-1.));
#41017=DIRECTION('ref_axis',(5.00596043936355E-16,1.,5.94374044734015E-16));
#41018=DIRECTION('',(-3.34404360992166E-15,5.94374044734026E-16,-1.));
#41019=DIRECTION('center_axis',(3.34404360992166E-15,-5.94374044734026E-16,
1.));
#41020=DIRECTION('ref_axis',(-5.00596043936355E-16,-1.,-5.94374044734015E-16));
#41021=DIRECTION('center_axis',(3.34404360992166E-15,-5.94374044734026E-16,
1.));
#41022=DIRECTION('ref_axis',(-5.00596043936355E-16,-1.,-5.94374044734015E-16));
#41023=DIRECTION('center_axis',(-3.34404360992166E-15,1.22120854809198E-15,
-1.));
#41024=DIRECTION('ref_axis',(-5.00596043936357E-16,-1.,-1.22120854809206E-15));
#41025=DIRECTION('',(-1.92402545023304E-15,0.707106781186548,-0.707106781186547));
#41026=DIRECTION('center_axis',(-3.34404360992165E-15,1.4543884843594E-14,
-1.));
#41027=DIRECTION('ref_axis',(-5.00596043936402E-16,-1.,-1.45438848435941E-14));
#41028=DIRECTION('',(-1.92402545023302E-15,0.707106781186553,-0.707106781186542));
#41029=DIRECTION('center_axis',(-3.34404360992165E-15,1.4543884843594E-14,
-1.));
#41030=DIRECTION('ref_axis',(-5.00596043936402E-16,-1.,-1.45438848435941E-14));
#41031=DIRECTION('',(-1.92402545023302E-15,0.707106781186553,-0.707106781186542));
#41032=DIRECTION('center_axis',(-3.34404360992166E-15,1.22120854809198E-15,
-1.));
#41033=DIRECTION('ref_axis',(-5.00596043936357E-16,-1.,-1.22120854809206E-15));
#41034=DIRECTION('',(-1.92402545023304E-15,0.707106781186548,-0.707106781186547));
#41035=DIRECTION('center_axis',(5.00596043936355E-16,1.,5.94374044734026E-16));
#41036=DIRECTION('ref_axis',(1.,-5.00596043936353E-16,-3.34404360992166E-15));
#41037=DIRECTION('',(-3.34404360992166E-15,5.94374044734026E-16,-1.));
#41038=DIRECTION('center_axis',(1.,-5.00596043936353E-16,-3.34404360992166E-15));
#41039=DIRECTION('ref_axis',(-5.00596043936355E-16,-1.,-6.88301496270999E-16));
#41040=DIRECTION('center_axis',(-3.34404360992239E-15,-1.45135967092772E-12,
-1.));
#41041=DIRECTION('ref_axis',(-1.,5.00596043936353E-16,3.34404360992166E-15));
#41042=DIRECTION('',(-1.,5.00596043936353E-16,3.34404360992166E-15));
#41043=DIRECTION('',(5.00596043931499E-16,1.,-1.45135967092772E-12));
#41044=DIRECTION('',(1.,-5.00596043936353E-16,-3.34404360992166E-15));
#41045=DIRECTION('center_axis',(-5.00596043936355E-16,-1.,-6.19091582357991E-16));
#41046=DIRECTION('ref_axis',(-1.,5.00596043936353E-16,3.34404360992166E-15));
#41047=DIRECTION('',(-3.34404360992166E-15,6.19091582358092E-16,-1.));
#41048=DIRECTION('center_axis',(5.00596043936355E-16,1.,6.19091582357991E-16));
#41049=DIRECTION('ref_axis',(1.,-5.00596043936353E-16,-3.34404360992166E-15));
#41050=DIRECTION('',(-3.34404360992166E-15,6.19091582358092E-16,-1.));
#41051=DIRECTION('center_axis',(1.,-5.00596043936353E-16,-3.34404360992166E-15));
#41052=DIRECTION('ref_axis',(-5.00596043936355E-16,-1.,-6.88301496270999E-16));
#41053=DIRECTION('center_axis',(-1.,5.00596043936353E-16,3.34404360992166E-15));
#41054=DIRECTION('ref_axis',(5.00596043936355E-16,1.,6.88301496270999E-16));
#41055=DIRECTION('',(-5.00596043931499E-16,-1.,1.45135967092772E-12));
#41056=DIRECTION('',(-3.34404360992166E-15,5.94374044734026E-16,-1.));
#41057=DIRECTION('center_axis',(5.00596043936355E-16,1.,5.94374044734026E-16));
#41058=DIRECTION('ref_axis',(1.,-5.00596043936353E-16,-3.34404360992166E-15));
#41059=DIRECTION('',(-1.,5.00596043936353E-16,3.34404360992166E-15));
#41060=DIRECTION('center_axis',(-3.34404360992239E-15,-1.45135967092772E-12,
-1.));
#41061=DIRECTION('ref_axis',(-1.,5.00596043936353E-16,3.34404360992166E-15));
#41062=DIRECTION('center_axis',(-3.34404360992239E-15,-1.45135967092772E-12,
-1.));
#41063=DIRECTION('ref_axis',(-1.,5.00596043936353E-16,3.34404360992166E-15));
#41064=DIRECTION('',(1.,-5.00596043936353E-16,-3.34404360992166E-15));
#41065=DIRECTION('center_axis',(-5.00596043936355E-16,-1.,-6.19091582356982E-16));
#41066=DIRECTION('ref_axis',(-1.,5.00596043936353E-16,3.34404360992166E-15));
#41067=DIRECTION('center_axis',(-5.00596043936355E-16,-1.,-6.19091607820957E-16));
#41068=DIRECTION('ref_axis',(-1.,5.00596043936353E-16,3.34404360992166E-15));
#41069=DIRECTION('',(3.34404360992166E-15,-6.19091607821058E-16,1.));
#41070=DIRECTION('',(-3.34404360992166E-15,6.19091607821058E-16,-1.));
#41071=DIRECTION('center_axis',(1.,-5.00596043936353E-16,-3.34404360992166E-15));
#41072=DIRECTION('ref_axis',(-5.00596043936355E-16,-1.,-6.88301496270999E-16));
#41073=DIRECTION('',(3.34404360992166E-15,-6.19091607821058E-16,1.));
#41074=DIRECTION('center_axis',(5.00596043936355E-16,1.,6.19091607820957E-16));
#41075=DIRECTION('ref_axis',(1.,-5.00596043936353E-16,-3.34404360992166E-15));
#41076=DIRECTION('',(3.34404360992166E-15,-6.19091607821058E-16,1.));
#41077=DIRECTION('center_axis',(-1.,5.00596043936353E-16,3.34404360992166E-15));
#41078=DIRECTION('ref_axis',(5.00596043936355E-16,1.,6.88301496270999E-16));
#53354=CARTESIAN_POINT('',(0.,0.,0.));
#53355=CARTESIAN_POINT('Origin',(144.115917770964,-309.972007268788,340.708039952219));
#53356=CARTESIAN_POINT('',(184.115917770964,-310.472007268788,340.708039952219));
#53357=CARTESIAN_POINT('',(184.115917770964,-309.972007268788,340.208039952218));
#53358=CARTESIAN_POINT('Origin',(184.115917770964,-309.972007268788,340.708039952219));
#53359=CARTESIAN_POINT('',(454.11591777097,-309.972007268788,340.208039952218));
#53360=CARTESIAN_POINT('',(144.115917770964,-309.972007268788,340.208039952219));
#53361=CARTESIAN_POINT('',(454.11591777097,-310.472007268788,340.708039952218));
#53362=CARTESIAN_POINT('Origin',(454.11591777097,-309.972007268788,340.708039952218));
#53363=CARTESIAN_POINT('',(144.115917770964,-310.472007268788,340.708039952219));
#53364=CARTESIAN_POINT('Origin',(144.115917770964,-310.472007268788,340.208039952219));
#53365=CARTESIAN_POINT('',(184.115917770964,-270.472007268788,340.208039952219));
#53366=CARTESIAN_POINT('',(184.115917770964,-290.472007268788,340.208039952219));
#53367=CARTESIAN_POINT('',(144.615917770964,-270.472007268788,340.208039952219));
#53368=CARTESIAN_POINT('',(144.115917770964,-270.472007268788,340.208039952219));
#53369=CARTESIAN_POINT('',(144.615917770964,-10.7242208197787,340.208039952219));
#53370=CARTESIAN_POINT('',(144.615917770964,-150.084339619182,340.208039952219));
#53371=CARTESIAN_POINT('',(184.115917770964,-10.7242208197787,340.208039952219));
#53372=CARTESIAN_POINT('',(164.115917770964,-10.7242208197787,340.208039952219));
#53373=CARTESIAN_POINT('',(184.115917770964,29.1607759831004,340.208039952219));
#53374=CARTESIAN_POINT('',(184.115917770964,-140.598114044284,340.208039952219));
#53375=CARTESIAN_POINT('',(454.11591777097,29.1607759831002,340.208039952218));
#53376=CARTESIAN_POINT('',(144.115917770964,29.1607759831004,340.208039952219));
#53377=CARTESIAN_POINT('',(454.11591777097,-10.7242208197788,340.208039952218));
#53378=CARTESIAN_POINT('',(454.11591777097,-160.598114044284,340.208039952218));
#53379=CARTESIAN_POINT('',(493.61591777097,-10.7242208197789,340.208039952218));
#53380=CARTESIAN_POINT('',(319.115917770967,-10.7242208197788,340.208039952218));
#53381=CARTESIAN_POINT('',(493.61591777097,-270.472007268782,340.208039952218));
#53382=CARTESIAN_POINT('',(493.61591777097,-150.222007268789,340.208039952218));
#53383=CARTESIAN_POINT('',(454.11591777097,-270.472007268782,340.208039952218));
#53384=CARTESIAN_POINT('',(299.115917770967,-270.472007268782,340.208039952218));
#53385=CARTESIAN_POINT('',(454.11591777097,-310.472007268785,340.208039952218));
#53386=CARTESIAN_POINT('',(444.115917770964,-64.2840072687828,340.208039952218));
#53387=CARTESIAN_POINT('Origin',(444.115917770964,-70.4720072687828,340.208039952218));
#53388=CARTESIAN_POINT('',(194.115917770964,-284.284007268782,340.208039952219));
#53389=CARTESIAN_POINT('Origin',(194.115917770964,-290.472007268782,340.208039952219));
#53390=CARTESIAN_POINT('',(444.115917770964,-100.472007268783,340.208039952218));
#53391=CARTESIAN_POINT('',(194.115917770964,-100.472007268783,340.208039952219));
#53392=CARTESIAN_POINT('',(169.115917770964,-100.472007268783,340.208039952219));
#53393=CARTESIAN_POINT('',(194.115917770964,-260.472007268782,340.208039952219));
#53394=CARTESIAN_POINT('',(194.115917770964,-285.472007268785,340.208039952219));
#53395=CARTESIAN_POINT('',(444.115917770964,-260.472007268782,340.208039952218));
#53396=CARTESIAN_POINT('',(294.115917770964,-260.472007268782,340.208039952218));
#53397=CARTESIAN_POINT('',(444.115917770964,-205.472007268785,340.208039952218));
#53398=CARTESIAN_POINT('',(194.115917770964,-64.2840072687827,340.208039952219));
#53399=CARTESIAN_POINT('Origin',(194.115917770964,-70.4720072687827,340.208039952219));
#53400=CARTESIAN_POINT('',(444.115917770964,-284.284007268782,340.208039952218));
#53401=CARTESIAN_POINT('Origin',(444.115917770964,-290.472007268782,340.208039952218));
#53402=CARTESIAN_POINT('Origin',(493.61591777097,-150.222007268789,340.708039952218));
#53403=CARTESIAN_POINT('',(494.11591777097,-10.7242208197795,340.708039952218));
#53404=CARTESIAN_POINT('Origin',(493.61591777097,-10.7242208197795,340.708039952218));
#53405=CARTESIAN_POINT('',(494.11591777097,-270.472007268782,340.708039952217));
#53406=CARTESIAN_POINT('',(494.11591777097,-150.222007268789,340.708039952218));
#53407=CARTESIAN_POINT('Origin',(493.61591777097,-270.472007268782,340.708039952217));
#53408=CARTESIAN_POINT('Origin',(494.11591777097,10.0279927312103,335.389856654884));
#53409=CARTESIAN_POINT('',(494.11591777097,-270.472007268782,320.779712758553));
#53410=CARTESIAN_POINT('',(494.11591777097,-270.472007268782,340.208039952218));
#53411=CARTESIAN_POINT('',(494.11591777097,-10.7242208197793,320.779712758176));
#53412=CARTESIAN_POINT('',(494.11591777097,-10.7242208197789,340.208039952218));
#53413=CARTESIAN_POINT('',(494.11591777097,29.2757791802208,320.779712758118));
#53414=CARTESIAN_POINT('',(494.11591777097,-55.6611674320453,320.779712758241));
#53415=CARTESIAN_POINT('',(494.11591777097,29.2757791802205,340.763897945769));
#53416=CARTESIAN_POINT('',(494.11591777097,29.2757791802212,340.208039952218));
#53417=CARTESIAN_POINT('',(494.11591777097,69.3907823772571,321.27971275806));
#53418=CARTESIAN_POINT('',(494.11591777097,22.6541183795134,343.980092760897));
#53419=CARTESIAN_POINT('',(494.11591777097,330.027992731203,321.279712757682));
#53420=CARTESIAN_POINT('',(494.11591777097,39.6518859556631,321.279712758103));
#53421=CARTESIAN_POINT('',(494.11591777097,330.027992731208,330.071673357551));
#53422=CARTESIAN_POINT('',(494.11591777097,330.027992731207,328.084784706188));
#53423=CARTESIAN_POINT('',(494.11591777097,71.6429959273593,330.071673357978));
#53424=CARTESIAN_POINT('',(494.11591777097,170.277992731204,330.071673357815));
#53425=CARTESIAN_POINT('',(494.11591777097,71.2060964085143,330.172163040955));
#53426=CARTESIAN_POINT('Origin',(494.11591777097,71.6429959273607,331.071673357978));
#53427=CARTESIAN_POINT('',(494.11591777097,31.4129895340987,349.500000551885));
#53428=CARTESIAN_POINT('',(494.11591777097,45.4823770730766,342.666383938589));
#53429=CARTESIAN_POINT('',(494.11591777097,-309.972007268783,349.500000552087));
#53430=CARTESIAN_POINT('',(494.11591777097,20.7779927312187,349.500000551892));
#53431=CARTESIAN_POINT('',(494.11591777097,-309.9720072688,320.77971275861));
#53432=CARTESIAN_POINT('',(494.11591777097,-309.972007268787,342.694928603579));
#53433=CARTESIAN_POINT('',(494.11591777097,-205.535060656547,320.779712758459));
#53434=CARTESIAN_POINT('Origin',(144.115917770964,29.1607759831001,339.708039952219));
#53435=CARTESIAN_POINT('',(454.11591777097,29.2757791802212,340.194634511016));
#53436=CARTESIAN_POINT('Origin',(454.11591777097,29.1607759830999,339.708039952218));
#53437=CARTESIAN_POINT('',(184.115917770964,29.2757791802213,340.194634511017));
#53438=CARTESIAN_POINT('Origin',(184.115917770964,29.1607759831001,339.708039952219));
#53439=CARTESIAN_POINT('',(184.115917770964,29.3792257425212,340.157795110731));
#53440=CARTESIAN_POINT('Origin',(184.115917770964,29.1607759831001,339.708039952219));
#53441=CARTESIAN_POINT('',(454.11591777097,29.3792257425211,340.15779511073));
#53442=CARTESIAN_POINT('',(144.115917770964,29.3792257425212,340.157795110731));
#53443=CARTESIAN_POINT('Origin',(454.11591777097,29.1607759830999,339.708039952218));
#53444=CARTESIAN_POINT('Ctrl Pts',(184.00935480449,29.1751198286203,340.231155563991));
#53445=CARTESIAN_POINT('Ctrl Pts',(184.035423606558,29.2301677887044,340.211275129548));
#53446=CARTESIAN_POINT('Ctrl Pts',(184.073633409372,29.2757791802213,340.194634511017));
#53447=CARTESIAN_POINT('Ctrl Pts',(184.115917770964,29.2757791802213,340.194634511017));
#53448=CARTESIAN_POINT('Ctrl Pts',(183.973228480221,29.2110507307293,340.230753219288));
#53449=CARTESIAN_POINT('Ctrl Pts',(184.008848284769,29.2659644027493,340.206430896902));
#53450=CARTESIAN_POINT('Ctrl Pts',(184.05978698227,29.3114732703414,340.186198464193));
#53451=CARTESIAN_POINT('Ctrl Pts',(184.115917770964,29.3114732703414,340.186198464193));
#53452=CARTESIAN_POINT('Ctrl Pts',(183.935350991415,29.2451273482303,340.222927797744));
#53453=CARTESIAN_POINT('Ctrl Pts',(183.981473610584,29.3004359815563,340.196056293685));
#53454=CARTESIAN_POINT('Ctrl Pts',(184.045598704041,29.3462340025403,340.173819468708));
#53455=CARTESIAN_POINT('Ctrl Pts',(184.115917770964,29.3462340025403,340.173819468708));
#53456=CARTESIAN_POINT('Ctrl Pts',(183.89746801131,29.2757791799883,340.208039952332));
#53457=CARTESIAN_POINT('Ctrl Pts',(183.954098540875,29.3324097096283,340.180534040856));
#53458=CARTESIAN_POINT('Ctrl Pts',(184.031409794092,29.3792257425212,340.157795110731));
#53459=CARTESIAN_POINT('Ctrl Pts',(184.115917770964,29.3792257425212,340.157795110731));
#53460=CARTESIAN_POINT('',(183.897468011221,29.2757791800603,340.208039952297));
#53461=CARTESIAN_POINT('Ctrl Pts',(183.897468011543,29.2757791802213,340.208039952219));
#53462=CARTESIAN_POINT('Ctrl Pts',(183.940017338202,29.2757791802213,340.208039952219));
#53463=CARTESIAN_POINT('Ctrl Pts',(183.980384153199,29.2757791801524,340.204672075941));
#53464=CARTESIAN_POINT('Ctrl Pts',(184.03989064397,29.2757791801524,340.199197864216));
#53465=CARTESIAN_POINT('Ctrl Pts',(184.061235828154,29.2757791802213,340.197088039368));
#53466=CARTESIAN_POINT('Ctrl Pts',(184.08771011489,29.2757791802213,340.195413965406));
#53467=CARTESIAN_POINT('Ctrl Pts',(184.094309573317,29.2757791802213,340.195080500941));
#53468=CARTESIAN_POINT('Ctrl Pts',(184.105942202007,29.2757791802213,340.194717028763));
#53469=CARTESIAN_POINT('Ctrl Pts',(184.110902933059,29.2757791802213,340.194634511017));
#53470=CARTESIAN_POINT('Ctrl Pts',(184.115917770964,29.2757791802213,340.194634511017));
#53471=CARTESIAN_POINT('Origin',(184.115917770914,28.3498010374177,340.657795110545));
#53472=CARTESIAN_POINT('Ctrl Pts',(454.11591777097,29.2757791802212,340.194634511016));
#53473=CARTESIAN_POINT('Ctrl Pts',(454.158236522942,29.2757791802212,340.194634511016));
#53474=CARTESIAN_POINT('Ctrl Pts',(454.196425407472,29.2301393405342,340.211285403533));
#53475=CARTESIAN_POINT('Ctrl Pts',(454.222480737526,29.1751198284492,340.231155564052));
#53476=CARTESIAN_POINT('Ctrl Pts',(454.11591777097,29.3114732703412,340.186198464192));
#53477=CARTESIAN_POINT('Ctrl Pts',(454.17209421151,29.3114732703412,340.186198464192));
#53478=CARTESIAN_POINT('Ctrl Pts',(454.223005665121,29.2659360239782,340.206443466406));
#53479=CARTESIAN_POINT('Ctrl Pts',(454.258607061825,29.2110507305572,340.230753219363));
#53480=CARTESIAN_POINT('Ctrl Pts',(454.11591777097,29.3462340025402,340.173819468707));
#53481=CARTESIAN_POINT('Ctrl Pts',(454.186294029236,29.3462340025402,340.173819468707));
#53482=CARTESIAN_POINT('Ctrl Pts',(454.250385767052,29.3004073986722,340.196070180577));
#53483=CARTESIAN_POINT('Ctrl Pts',(454.296484550663,29.2451273480572,340.222927797827));
#53484=CARTESIAN_POINT('Ctrl Pts',(454.11591777097,29.3792257425211,340.15779511073));
#53485=CARTESIAN_POINT('Ctrl Pts',(454.200494479196,29.3792257425211,340.15779511073));
#53486=CARTESIAN_POINT('Ctrl Pts',(454.27776626714,29.3323804436042,340.180548255603));
#53487=CARTESIAN_POINT('Ctrl Pts',(454.334367530801,29.2757791798112,340.208039952417));
#53488=CARTESIAN_POINT('',(454.334367530957,29.2757791799382,340.208039952355));
#53489=CARTESIAN_POINT('Ctrl Pts',(454.11591777097,29.2757791802212,340.194634511016));
#53490=CARTESIAN_POINT('Ctrl Pts',(454.120938618672,29.2757791802212,340.194634511016));
#53491=CARTESIAN_POINT('Ctrl Pts',(454.125905101463,29.2757791802212,340.194717142149));
#53492=CARTESIAN_POINT('Ctrl Pts',(454.137553824068,29.2757791802212,340.195081275641));
#53493=CARTESIAN_POINT('Ctrl Pts',(454.144163062791,29.2757791802211,340.19541545435));
#53494=CARTESIAN_POINT('Ctrl Pts',(454.171630390795,29.2757791802211,340.197153487144));
#53495=CARTESIAN_POINT('Ctrl Pts',(454.190169235585,29.2757791802179,340.199034540506));
#53496=CARTESIAN_POINT('Ctrl Pts',(454.251614129388,29.2757791802179,340.204685275396));
#53497=CARTESIAN_POINT('Ctrl Pts',(454.291901888822,29.2757791802212,340.208039952218));
#53498=CARTESIAN_POINT('Ctrl Pts',(454.334367530392,29.2757791802212,340.208039952218));
#53499=CARTESIAN_POINT('Origin',(454.115917771007,28.3498010373495,340.657795110577));
#53500=CARTESIAN_POINT('Origin',(454.11591777097,-10.7242208197788,340.208039952218));
#53501=CARTESIAN_POINT('',(454.11591777097,29.2757791802208,320.779712758118));
#53502=CARTESIAN_POINT('',(454.11591777097,29.2757791802212,340.208039952218));
#53503=CARTESIAN_POINT('',(454.11591777097,-10.7242208197793,320.779712758176));
#53504=CARTESIAN_POINT('',(454.11591777097,-75.6611674320453,320.77971275827));
#53505=CARTESIAN_POINT('',(454.11591777097,-10.7242208197788,340.208039952218));
#53506=CARTESIAN_POINT('Origin',(454.11591777097,29.2757791802212,340.208039952218));
#53507=CARTESIAN_POINT('',(493.61591777097,29.2757791802212,340.208039952218));
#53508=CARTESIAN_POINT('',(144.115917770964,29.2757791802213,340.208039952219));
#53509=CARTESIAN_POINT('Origin',(493.61591777097,29.2757791802205,340.763897945769));
#53510=CARTESIAN_POINT('',(386.615917770969,29.2757791802208,320.779712758118));
#53511=CARTESIAN_POINT('Origin',(144.115917770964,29.2757791802213,340.208039952219));
#53512=CARTESIAN_POINT('',(144.615917770964,29.2757791802213,340.208039952219));
#53513=CARTESIAN_POINT('',(144.115917770964,29.2757791802213,340.208039952219));
#53514=CARTESIAN_POINT('',(144.615917770964,69.1723326178359,320.829957599548));
#53515=CARTESIAN_POINT('',(144.615917770964,22.3118351489324,343.590484532268));
#53516=CARTESIAN_POINT('',(493.61591777097,69.1723326178358,320.829957599547));
#53517=CARTESIAN_POINT('',(144.115917770964,69.1723326178359,320.829957599548));
#53518=CARTESIAN_POINT('',(493.61591777097,22.4356686200921,343.530337602384));
#53519=CARTESIAN_POINT('Origin',(144.615917770964,-150.084339619182,340.708039952219));
#53520=CARTESIAN_POINT('',(144.115917770964,-10.7242208197794,340.708039952219));
#53521=CARTESIAN_POINT('Origin',(144.615917770964,-10.7242208197794,340.708039952219));
#53522=CARTESIAN_POINT('',(144.115917770964,-270.472007268788,340.708039952219));
#53523=CARTESIAN_POINT('Origin',(144.615917770964,-270.472007268788,340.708039952219));
#53524=CARTESIAN_POINT('',(144.115917770964,-150.084339619182,340.708039952219));
#53525=CARTESIAN_POINT('Origin',(144.615917770964,69.3907823772572,321.279712758061));
#53526=CARTESIAN_POINT('',(144.115917770964,69.3907823772572,321.279712758061));
#53527=CARTESIAN_POINT('Origin',(144.615917770964,69.3907823772572,321.279712758061));
#53528=CARTESIAN_POINT('',(144.615917770964,69.3907823772569,320.779712758061));
#53529=CARTESIAN_POINT('Origin',(144.615917770964,69.3907823772572,321.279712758061));
#53530=CARTESIAN_POINT('Origin',(144.615917770964,69.3907823772572,321.279712758061));
#53531=CARTESIAN_POINT('Origin',(493.61591777097,69.3907823772571,321.27971275806));
#53532=CARTESIAN_POINT('',(493.61591777097,69.3907823772568,320.77971275806));
#53533=CARTESIAN_POINT('Origin',(493.61591777097,69.3907823772571,321.27971275806));
#53534=CARTESIAN_POINT('Origin',(493.61591777097,69.3907823772571,321.27971275806));
#53535=CARTESIAN_POINT('Origin',(493.61591777097,69.3907823772571,321.27971275806));
#53536=CARTESIAN_POINT('Origin',(144.615917770964,330.027992731203,321.279712757683));
#53537=CARTESIAN_POINT('',(144.115917770964,330.027992731203,321.279712757683));
#53538=CARTESIAN_POINT('',(144.615917770964,330.027992731203,320.779712757683));
#53539=CARTESIAN_POINT('Origin',(144.615917770964,330.027992731203,321.279712757683));
#53540=CARTESIAN_POINT('',(144.615917770964,330.527992731203,321.279712757682));
#53541=CARTESIAN_POINT('Origin',(144.615917770964,330.027992731203,321.279712757683));
#53542=CARTESIAN_POINT('Origin',(144.615917770964,330.027992731203,321.279712757683));
#53543=CARTESIAN_POINT('Origin',(493.61591777097,330.027992731203,321.279712757682));
#53544=CARTESIAN_POINT('',(493.61591777097,330.527992731203,321.279712757681));
#53545=CARTESIAN_POINT('',(493.61591777097,330.027992731203,320.779712757682));
#53546=CARTESIAN_POINT('Origin',(493.61591777097,330.027992731203,321.279712757682));
#53547=CARTESIAN_POINT('Origin',(493.61591777097,330.027992731203,321.279712757682));
#53548=CARTESIAN_POINT('Origin',(493.61591777097,330.027992731203,321.279712757682));
#53549=CARTESIAN_POINT('Origin',(144.615917770964,330.027992731208,330.071673357552));
#53550=CARTESIAN_POINT('',(144.115917770964,330.027992731208,330.071673357552));
#53551=CARTESIAN_POINT('',(144.615917770964,330.527992731208,330.071673357552));
#53552=CARTESIAN_POINT('Origin',(144.615917770964,330.027992731208,330.071673357552));
#53553=CARTESIAN_POINT('',(144.615917770964,330.027992731209,330.571673357552));
#53554=CARTESIAN_POINT('Origin',(144.615917770964,330.027992731208,330.071673357552));
#53555=CARTESIAN_POINT('Origin',(144.615917770964,330.027992731208,330.071673357552));
#53556=CARTESIAN_POINT('Origin',(493.61591777097,330.027992731208,330.071673357551));
#53557=CARTESIAN_POINT('',(493.61591777097,330.027992731208,330.571673357551));
#53558=CARTESIAN_POINT('',(493.61591777097,330.527992731208,330.071673357551));
#53559=CARTESIAN_POINT('Origin',(493.61591777097,330.027992731208,330.071673357551));
#53560=CARTESIAN_POINT('Origin',(493.61591777097,330.027992731208,330.071673357551));
#53561=CARTESIAN_POINT('Origin',(493.61591777097,330.027992731208,330.071673357551));
#53562=CARTESIAN_POINT('Origin',(144.615917770964,71.6429959273609,331.071673357979));
#53563=CARTESIAN_POINT('',(144.115917770964,71.6429959273594,330.071673357979));
#53564=CARTESIAN_POINT('',(144.115917770964,71.2060964085144,330.172163040956));
#53565=CARTESIAN_POINT('Origin',(144.115917770964,71.6429959273609,331.07167335798));
#53566=CARTESIAN_POINT('',(144.615917770964,71.4245461679377,330.621918199468));
#53567=CARTESIAN_POINT('Origin',(144.615917770964,71.2060964085144,330.172163040956));
#53568=CARTESIAN_POINT('',(144.615917770964,71.6429959273606,330.571673357979));
#53569=CARTESIAN_POINT('Origin',(144.615917770964,71.6429959273609,331.071673357979));
#53570=CARTESIAN_POINT('Origin',(144.615917770964,71.6429959273594,330.071673357979));
#53571=CARTESIAN_POINT('Origin',(493.61591777097,71.6429959273607,331.071673357978));
#53572=CARTESIAN_POINT('',(493.61591777097,71.4245461679375,330.621918199467));
#53573=CARTESIAN_POINT('',(493.61591777097,71.6429959273605,330.571673357978));
#53574=CARTESIAN_POINT('Origin',(493.61591777097,71.6429959273607,331.071673357978));
#53575=CARTESIAN_POINT('Origin',(493.61591777097,71.2060964085143,330.172163040955));
#53576=CARTESIAN_POINT('Origin',(493.61591777097,71.6429959273593,330.071673357978));
#53577=CARTESIAN_POINT('Origin',(144.615917770964,31.4129895340988,349.500000551887));
#53578=CARTESIAN_POINT('',(144.115917770964,31.4129895340988,349.500000551887));
#53579=CARTESIAN_POINT('',(144.615917770964,31.6314392935211,349.949755710398));
#53580=CARTESIAN_POINT('Origin',(144.615917770964,31.4129895340988,349.500000551887));
#53581=CARTESIAN_POINT('',(144.615917770964,31.4129895340991,350.000000551887));
#53582=CARTESIAN_POINT('Origin',(144.615917770964,31.4129895340988,349.500000551887));
#53583=CARTESIAN_POINT('Origin',(144.615917770964,31.4129895340988,349.500000551887));
#53584=CARTESIAN_POINT('Origin',(144.615917770964,-309.972007268782,349.500000552088));
#53585=CARTESIAN_POINT('',(144.615917770964,-309.972007268782,350.000000552088));
#53586=CARTESIAN_POINT('',(144.615917770964,-310.472007268782,349.500000552088));
#53587=CARTESIAN_POINT('Origin',(144.615917770964,-309.972007268782,349.500000552088));
#53588=CARTESIAN_POINT('',(144.115917770964,-309.972007268782,349.500000552088));
#53589=CARTESIAN_POINT('Origin',(144.615917770964,-309.972007268782,349.500000552088));
#53590=CARTESIAN_POINT('Origin',(144.615917770964,-309.972007268782,349.500000552088));
#53591=CARTESIAN_POINT('Origin',(144.615917770964,20.9156603808258,349.500000551893));
#53592=CARTESIAN_POINT('',(144.115917770964,20.9156603808258,349.500000551893));
#53593=CARTESIAN_POINT('',(144.615917770964,20.9156603808261,350.000000551893));
#53594=CARTESIAN_POINT('Origin',(144.615917770964,-309.972007268786,343.293466961922));
#53595=CARTESIAN_POINT('',(144.115917770964,-309.972007268799,320.779712758612));
#53596=CARTESIAN_POINT('',(144.615917770964,-310.472007268788,320.779712758612));
#53597=CARTESIAN_POINT('Origin',(144.615917770964,-309.972007268799,320.779712758466));
#53598=CARTESIAN_POINT('',(144.615917770964,-310.472007268786,343.293466961922));
#53599=CARTESIAN_POINT('',(144.115917770964,-309.972007268786,343.293466961922));
#53600=CARTESIAN_POINT('Origin',(493.61591777097,31.4129895340987,349.500000551885));
#53601=CARTESIAN_POINT('',(493.61591777097,31.412989534099,350.000000551885));
#53602=CARTESIAN_POINT('Origin',(493.61591777097,31.4129895340987,349.500000551885));
#53603=CARTESIAN_POINT('',(493.61591777097,31.6314392935209,349.949755710397));
#53604=CARTESIAN_POINT('Origin',(493.61591777097,31.4129895340987,349.500000551885));
#53605=CARTESIAN_POINT('Origin',(493.61591777097,31.4129895340987,349.500000551885));
#53606=CARTESIAN_POINT('Origin',(493.61591777097,45.4823770730766,342.666383938589));
#53607=CARTESIAN_POINT('',(493.61591777097,45.7008268324999,343.116139097101));
#53608=CARTESIAN_POINT('Origin',(144.115917770964,31.4129895340988,349.500000551887));
#53609=CARTESIAN_POINT('',(144.115917770964,31.6314392935211,349.949755710398));
#53610=CARTESIAN_POINT('',(144.115917770964,31.4129895340991,350.000000551887));
#53611=CARTESIAN_POINT('Origin',(493.61591777097,-309.972007268783,349.500000552087));
#53612=CARTESIAN_POINT('',(493.61591777097,-310.472007268783,349.500000552087));
#53613=CARTESIAN_POINT('',(493.61591777097,-309.972007268782,350.000000552087));
#53614=CARTESIAN_POINT('Origin',(493.61591777097,-309.972007268783,349.500000552087));
#53615=CARTESIAN_POINT('Origin',(493.61591777097,-309.972007268783,349.500000552087));
#53616=CARTESIAN_POINT('Origin',(493.61591777097,-309.972007268783,349.500000552087));
#53617=CARTESIAN_POINT('Origin',(493.61591777097,-309.972007268787,342.694928603579));
#53618=CARTESIAN_POINT('',(493.61591777097,-310.472007268788,320.779712758611));
#53619=CARTESIAN_POINT('Origin',(493.61591777097,-309.9720072688,320.779712758464));
#53620=CARTESIAN_POINT('',(493.61591777097,-310.472007268787,342.69492860358));
#53621=CARTESIAN_POINT('Origin',(493.61591777097,20.7779927312187,349.500000551892));
#53622=CARTESIAN_POINT('',(493.61591777097,20.7779927312189,350.000000551892));
#53623=CARTESIAN_POINT('Origin',(144.115917770964,-309.972007268782,349.500000552088));
#53624=CARTESIAN_POINT('',(144.115917770964,-309.972007268782,350.000000552088));
#53625=CARTESIAN_POINT('',(144.115917770964,-310.472007268782,349.500000552088));
#53626=CARTESIAN_POINT('Origin',(144.615917770964,45.3585436019158,342.726530868474));
#53627=CARTESIAN_POINT('',(144.115917770964,45.3585436019158,342.726530868474));
#53628=CARTESIAN_POINT('',(144.615917770964,45.576993361338,343.176286026986));
#53629=CARTESIAN_POINT('Origin',(493.61591777097,170.277992731204,330.071673357815));
#53630=CARTESIAN_POINT('',(493.61591777097,170.277992731206,330.571673357815));
#53631=CARTESIAN_POINT('Origin',(144.115917770964,71.6429959273609,331.071673357979));
#53632=CARTESIAN_POINT('',(144.115917770964,71.6429959273606,330.571673357979));
#53633=CARTESIAN_POINT('',(144.115917770964,71.4245461679377,330.621918199468));
#53634=CARTESIAN_POINT('Origin',(144.615917770964,170.41566038081,330.071673357816));
#53635=CARTESIAN_POINT('',(144.115917770964,170.41566038081,330.071673357816));
#53636=CARTESIAN_POINT('',(144.615917770964,170.415660380812,330.571673357816));
#53637=CARTESIAN_POINT('Origin',(493.61591777097,330.027992731207,328.084784706188));
#53638=CARTESIAN_POINT('',(493.61591777097,330.527992731207,328.084784706188));
#53639=CARTESIAN_POINT('Origin',(144.115917770964,330.027992731208,330.071673357552));
#53640=CARTESIAN_POINT('',(144.115917770964,330.527992731208,330.071673357552));
#53641=CARTESIAN_POINT('',(144.115917770964,330.027992731209,330.571673357552));
#53642=CARTESIAN_POINT('Origin',(144.615917770964,330.027992731207,328.683323064531));
#53643=CARTESIAN_POINT('',(144.115917770964,330.027992731207,328.683323064531));
#53644=CARTESIAN_POINT('',(144.615917770964,330.527992731208,328.68332306453));
#53645=CARTESIAN_POINT('Origin',(493.61591777097,39.6518859556631,321.279712758103));
#53646=CARTESIAN_POINT('',(493.61591777097,39.6518859556628,320.779712758103));
#53647=CARTESIAN_POINT('Origin',(144.115917770964,330.027992731203,321.279712757683));
#53648=CARTESIAN_POINT('',(144.115917770964,330.027992731203,320.779712757683));
#53649=CARTESIAN_POINT('',(144.115917770964,330.527992731203,321.279712757682));
#53650=CARTESIAN_POINT('Origin',(144.615917770964,39.7895536052691,321.279712758104));
#53651=CARTESIAN_POINT('',(144.115917770964,39.7895536052691,321.279712758104));
#53652=CARTESIAN_POINT('',(144.615917770964,39.7895536052689,320.779712758104));
#53653=CARTESIAN_POINT('Origin',(493.61591777097,22.6541183795134,343.980092760897));
#53654=CARTESIAN_POINT('Origin',(144.115917770964,69.3907823772572,321.279712758061));
#53655=CARTESIAN_POINT('',(144.115917770964,69.3907823772569,320.779712758061));
#53656=CARTESIAN_POINT('Origin',(144.615917770964,22.5302849083546,344.04023969078));
#53657=CARTESIAN_POINT('',(144.115917770964,29.2757791802206,340.76389794577));
#53658=CARTESIAN_POINT('Origin',(144.615917770964,29.2757791802206,340.76389794577));
#53659=CARTESIAN_POINT('',(144.115917770964,22.5302849083546,344.04023969078));
#53660=CARTESIAN_POINT('Origin',(144.115917770964,-310.472007268782,350.000000552088));
#53661=CARTESIAN_POINT('',(454.11591777097,-310.472007268782,320.779712758611));
#53662=CARTESIAN_POINT('',(454.11591777097,-310.472007268782,340.208039952218));
#53663=CARTESIAN_POINT('',(406.615917770957,-310.472007268775,320.779712758611));
#53664=CARTESIAN_POINT('',(184.115917770964,-310.472007268788,320.779712758612));
#53665=CARTESIAN_POINT('',(251.615917770966,-310.472007268788,320.779712758612));
#53666=CARTESIAN_POINT('',(184.115917770964,-310.472007268788,340.208039952219));
#53667=CARTESIAN_POINT('Origin',(319.115917770967,-140.598114044283,320.779712758365));
#53668=CARTESIAN_POINT('',(144.115917770964,-270.472007268788,320.779712758554));
#53669=CARTESIAN_POINT('',(144.115917770964,-225.53506065655,320.779712758489));
#53670=CARTESIAN_POINT('',(184.115917770964,-270.472007268788,320.779712758554));
#53671=CARTESIAN_POINT('',(231.615917770965,-270.472007268788,320.779712758554));
#53672=CARTESIAN_POINT('',(184.115917770964,-205.53506065655,320.77971275846));
#53673=CARTESIAN_POINT('Origin',(144.115917770964,10.3033280304242,336.586933371568));
#53674=CARTESIAN_POINT('',(144.115917770964,-270.472007268788,340.208039952219));
#53675=CARTESIAN_POINT('',(144.115917770964,29.2757791802209,320.779712758119));
#53676=CARTESIAN_POINT('',(144.115917770964,29.2757791802213,340.208039952219));
#53677=CARTESIAN_POINT('',(144.115917770964,-10.7242208197791,320.779712758177));
#53678=CARTESIAN_POINT('',(144.115917770964,-75.6611674320451,320.779712758272));
#53679=CARTESIAN_POINT('',(144.115917770964,-10.7242208197787,340.208039952219));
#53680=CARTESIAN_POINT('Origin',(144.115917770964,31.5279927312201,350.000000551886));
#53681=CARTESIAN_POINT('',(444.115917770964,-296.660007268781,350.000000552079));
#53682=CARTESIAN_POINT('Origin',(444.115917770964,-290.472007268782,350.000000552075));
#53683=CARTESIAN_POINT('',(194.115917770964,-76.660007268782,350.00000055195));
#53684=CARTESIAN_POINT('Origin',(194.115917770964,-70.472007268782,350.000000551946));
#53685=CARTESIAN_POINT('',(194.115917770964,-100.472007268782,350.000000551964));
#53686=CARTESIAN_POINT('',(444.115917770964,-100.472007268782,350.000000551963));
#53687=CARTESIAN_POINT('',(169.115917770964,-100.472007268782,350.000000551964));
#53688=CARTESIAN_POINT('',(444.115917770964,-260.472007268782,350.000000552058));
#53689=CARTESIAN_POINT('',(444.115917770964,-34.4720072687781,350.000000551924));
#53690=CARTESIAN_POINT('',(194.115917770964,-260.472007268782,350.000000552058));
#53691=CARTESIAN_POINT('',(294.115917770964,-260.472007268782,350.000000552058));
#53692=CARTESIAN_POINT('',(194.115917770964,-114.472007268778,350.000000551972));
#53693=CARTESIAN_POINT('',(194.115917770964,-296.660007268781,350.00000055208));
#53694=CARTESIAN_POINT('Origin',(194.115917770964,-290.472007268782,350.000000552076));
#53695=CARTESIAN_POINT('',(444.115917770964,-76.6600072687821,350.000000551949));
#53696=CARTESIAN_POINT('Origin',(444.115917770964,-70.4720072687821,350.000000551946));
#53697=CARTESIAN_POINT('Origin',(144.115917770964,71.5279927302396,330.57167335798));
#53698=CARTESIAN_POINT('Origin',(144.115917770964,330.527992731209,330.571673357551));
#53699=CARTESIAN_POINT('Origin',(144.115917770964,330.527992731203,320.779712757682));
#53700=CARTESIAN_POINT('Origin',(144.115917770964,69.2757791801369,320.779712758061));
#53701=CARTESIAN_POINT('Origin',(444.115917770964,-290.472007268782,349.500000551887));
#53702=CARTESIAN_POINT('',(444.115917770964,-295.660007268782,349.000000551699));
#53703=CARTESIAN_POINT('Origin',(444.115917770964,-290.472007268782,349.000000551699));
#53704=CARTESIAN_POINT('',(444.115917770964,-296.160007268782,349.50000055189));
#53705=CARTESIAN_POINT('Origin',(444.115917770964,-290.472007268782,355.858039952218));
#53706=CARTESIAN_POINT('',(444.115917770964,-295.660007268782,341.208039952218));
#53707=CARTESIAN_POINT('',(444.115917770964,-295.660007268782,355.858039952218));
#53708=CARTESIAN_POINT('',(444.115917770964,-285.284007268782,341.208039952218));
#53709=CARTESIAN_POINT('Origin',(444.115917770964,-290.472007268782,341.208039952218));
#53710=CARTESIAN_POINT('Origin',(444.115917770964,-290.472007268782,341.208039952218));
#53711=CARTESIAN_POINT('Origin',(444.115917770964,-70.4720072687823,349.500000551887));
#53712=CARTESIAN_POINT('',(444.115917770964,-75.6600072687826,349.000000551829));
#53713=CARTESIAN_POINT('Origin',(444.115917770964,-70.4720072687826,349.000000551829));
#53714=CARTESIAN_POINT('',(444.115917770964,-76.1600072687821,349.50000055189));
#53715=CARTESIAN_POINT('Origin',(444.115917770964,-70.4720072687826,355.858039952218));
#53716=CARTESIAN_POINT('',(444.115917770964,-75.6600072687826,341.208039952218));
#53717=CARTESIAN_POINT('',(444.115917770964,-75.6600072687826,355.858039952218));
#53718=CARTESIAN_POINT('',(444.115917770964,-65.2840072687832,341.208039952218));
#53719=CARTESIAN_POINT('Origin',(444.115917770964,-70.4720072687833,341.208039952218));
#53720=CARTESIAN_POINT('Origin',(444.115917770964,-70.4720072687833,341.208039952218));
#53721=CARTESIAN_POINT('Origin',(194.115917770964,-70.4720072687822,349.500000551888));
#53722=CARTESIAN_POINT('',(194.115917770964,-75.6600072687825,349.00000055183));
#53723=CARTESIAN_POINT('Origin',(194.115917770964,-70.4720072687825,349.00000055183));
#53724=CARTESIAN_POINT('',(194.115917770964,-76.160007268782,349.500000551891));
#53725=CARTESIAN_POINT('Origin',(194.115917770964,-70.4720072687825,355.858039952219));
#53726=CARTESIAN_POINT('',(194.115917770964,-75.6600072687825,341.208039952219));
#53727=CARTESIAN_POINT('',(194.115917770964,-75.6600072687825,355.858039952219));
#53728=CARTESIAN_POINT('',(194.115917770964,-65.2840072687831,341.208039952219));
#53729=CARTESIAN_POINT('Origin',(194.115917770964,-70.4720072687832,341.208039952219));
#53730=CARTESIAN_POINT('Origin',(194.115917770964,-70.4720072687832,341.208039952219));
#53731=CARTESIAN_POINT('Origin',(194.115917770964,-290.472007268782,349.500000551888));
#53732=CARTESIAN_POINT('',(194.115917770964,-295.660007268782,349.0000005517));
#53733=CARTESIAN_POINT('Origin',(194.115917770964,-290.472007268782,349.0000005517));
#53734=CARTESIAN_POINT('',(194.115917770964,-296.160007268782,349.500000551891));
#53735=CARTESIAN_POINT('Origin',(194.115917770964,-290.472007268782,355.858039952219));
#53736=CARTESIAN_POINT('',(194.115917770964,-295.660007268782,341.208039952219));
#53737=CARTESIAN_POINT('',(194.115917770964,-295.660007268782,355.858039952219));
#53738=CARTESIAN_POINT('',(194.115917770964,-285.284007268782,341.208039952218));
#53739=CARTESIAN_POINT('Origin',(194.115917770964,-290.472007268782,341.208039952219));
#53740=CARTESIAN_POINT('Origin',(194.115917770964,-290.472007268782,341.208039952219));
#53741=CARTESIAN_POINT('Origin',(444.115917770964,-290.472007268782,340.708039952218));
#53742=CARTESIAN_POINT('',(444.115917770964,-284.784007268782,340.708039952218));
#53743=CARTESIAN_POINT('Origin',(444.115917770964,-70.4720072687825,340.708039952218));
#53744=CARTESIAN_POINT('',(444.115917770964,-64.7840072687825,340.708039952218));
#53745=CARTESIAN_POINT('Origin',(194.115917770964,-70.4720072687824,340.708039952219));
#53746=CARTESIAN_POINT('',(194.115917770964,-64.7840072687824,340.708039952219));
#53747=CARTESIAN_POINT('Origin',(194.115917770964,-290.472007268782,340.708039952218));
#53748=CARTESIAN_POINT('',(194.115917770964,-284.784007268782,340.708039952218));
#53749=CARTESIAN_POINT('Origin',(144.115917770964,-270.472007268788,340.208039952219));
#53750=CARTESIAN_POINT('',(184.115917770964,-270.472007268788,340.208039952219));
#53751=CARTESIAN_POINT('Origin',(184.115917770964,-270.472007268788,340.208039952219));
#53752=CARTESIAN_POINT('Origin',(319.115917770967,-140.598114044283,320.779712758365));
#53753=CARTESIAN_POINT('',(184.115917770964,29.2757791802209,320.779712758119));
#53754=CARTESIAN_POINT('',(231.615917770966,29.2757791802208,320.779712758119));
#53755=CARTESIAN_POINT('',(184.115917770964,-10.7242208197792,320.779712758177));
#53756=CARTESIAN_POINT('',(184.115917770964,-55.6611674320452,320.779712758242));
#53757=CARTESIAN_POINT('',(251.615917770966,-10.7242208197792,320.779712758177));
#53758=CARTESIAN_POINT('Origin',(184.115917770964,-10.7242208197787,340.208039952219));
#53759=CARTESIAN_POINT('',(184.115917770964,-10.7242208197787,340.208039952219));
#53760=CARTESIAN_POINT('Origin',(144.115917770964,29.2757791802213,340.208039952219));
#53761=CARTESIAN_POINT('',(184.115917770964,29.2757791802213,340.208039952219));
#53762=CARTESIAN_POINT('Origin',(184.115917770964,29.2757791802213,340.208039952219));
#53763=CARTESIAN_POINT('Origin',(454.11591777097,-310.472007268782,340.208039952218));
#53764=CARTESIAN_POINT('',(454.11591777097,-270.472007268782,320.779712758553));
#53765=CARTESIAN_POINT('',(454.11591777097,-225.535060656547,320.779712758488));
#53766=CARTESIAN_POINT('',(454.11591777097,-270.472007268782,340.208039952218));
#53767=CARTESIAN_POINT('Origin',(454.11591777097,-270.472007268782,340.208039952218));
#53768=CARTESIAN_POINT('',(386.615917770969,-270.472007268782,320.779712758553));
#53769=CARTESIAN_POINT('Origin',(319.115917770967,-140.598114044283,320.779712758365));
#53770=CARTESIAN_POINT('Origin',(319.115917770967,-140.598114044283,320.779712758365));
#53771=CARTESIAN_POINT('',(406.615917770969,-10.7242208197793,320.779712758176));
#53772=CARTESIAN_POINT('Origin',(494.11591777097,-10.7242208197789,340.208039952218));
#53773=CARTESIAN_POINT('Origin',(444.115917770964,-260.472007268782,340.208039952218));
#53774=CARTESIAN_POINT('',(194.115917770964,-260.472007268782,340.208039952219));
#53775=CARTESIAN_POINT('',(444.115917770964,-260.472007268782,340.208039952218));
#53776=CARTESIAN_POINT('Origin',(444.115917770964,-100.472007268783,340.208039952218));
#53777=CARTESIAN_POINT('',(444.115917770964,-100.472007268783,340.208039952218));
#53778=CARTESIAN_POINT('Origin',(194.115917770964,-100.472007268783,340.208039952219));
#53779=CARTESIAN_POINT('',(194.115917770964,-100.472007268783,340.208039952219));
#53780=CARTESIAN_POINT('Origin',(194.115917770964,-260.472007268782,340.208039952219));
#61760=UNCERTAINTY_MEASURE_WITH_UNIT(LENGTH_MEASURE(0.01),#61812,
'DISTANCE_ACCURACY_VALUE',
'Maximum model space distance between geometric entities at asserted c
onnectivities');
#61780=UNCERTAINTY_MEASURE_WITH_UNIT(LENGTH_MEASURE(0.01),#61812,
'DISTANCE_ACCURACY_VALUE',
'Maximum model space distance between geometric entities at asserted c
onnectivities');
#61791=(
GEOMETRIC_REPRESENTATION_CONTEXT(3)
GLOBAL_UNCERTAINTY_ASSIGNED_CONTEXT((#61760))
GLOBAL_UNIT_ASSIGNED_CONTEXT((#61812,#61814,#61815))
REPRESENTATION_CONTEXT('','3D')
);
#61811=(
GEOMETRIC_REPRESENTATION_CONTEXT(3)
GLOBAL_UNCERTAINTY_ASSIGNED_CONTEXT((#61780))
GLOBAL_UNIT_ASSIGNED_CONTEXT((#61812,#61814,#61815))
REPRESENTATION_CONTEXT('','3D')
);
#61812=(
LENGTH_UNIT()
NAMED_UNIT(*)
SI_UNIT(.MILLI.,.METRE.)
);
#61814=(
NAMED_UNIT(*)
PLANE_ANGLE_UNIT()
SI_UNIT($,.RADIAN.)
);
#61815=(
NAMED_UNIT(*)
SI_UNIT($,.STERADIAN.)
SOLID_ANGLE_UNIT()
);
#61826=SHAPE_DEFINITION_REPRESENTATION(#61856,#61978);
#61856=PRODUCT_DEFINITION_SHAPE('',$,#62009);
#61978=SHAPE_REPRESENTATION('',(#35040),#61791);
#61998=PRODUCT_DEFINITION_CONTEXT('part definition',#62090,'design');
#62009=PRODUCT_DEFINITION('Motor and Gearbox Mounting Plate',
'Motor and Gearbox Mounting Plate',#62039,#61998);
#62039=PRODUCT_DEFINITION_FORMATION('',$,#62102);
#62090=APPLICATION_CONTEXT('Managed model based 3d engineering');
#62091=PRODUCT_CONTEXT('part definition',#62090,'mechanical');
#62102=PRODUCT('Motor and Gearbox Mounting Plate',
'Motor and Gearbox Mounting Plate',$,(#62091));
#62136=COLOUR_RGB('Light Blue',0.38,0.62,0.78);
#62137=FILL_AREA_STYLE_COLOUR('',#62136);
#62138=FILL_AREA_STYLE('',(#62137));
#62139=SURFACE_STYLE_FILL_AREA(#62138);
#62140=SURFACE_SIDE_STYLE('',(#62139));
#62141=SURFACE_STYLE_USAGE(.BOTH.,#62140);
#62142=PRESENTATION_STYLE_ASSIGNMENT((#62141));
ENDSEC;
END-ISO-10303-21;
